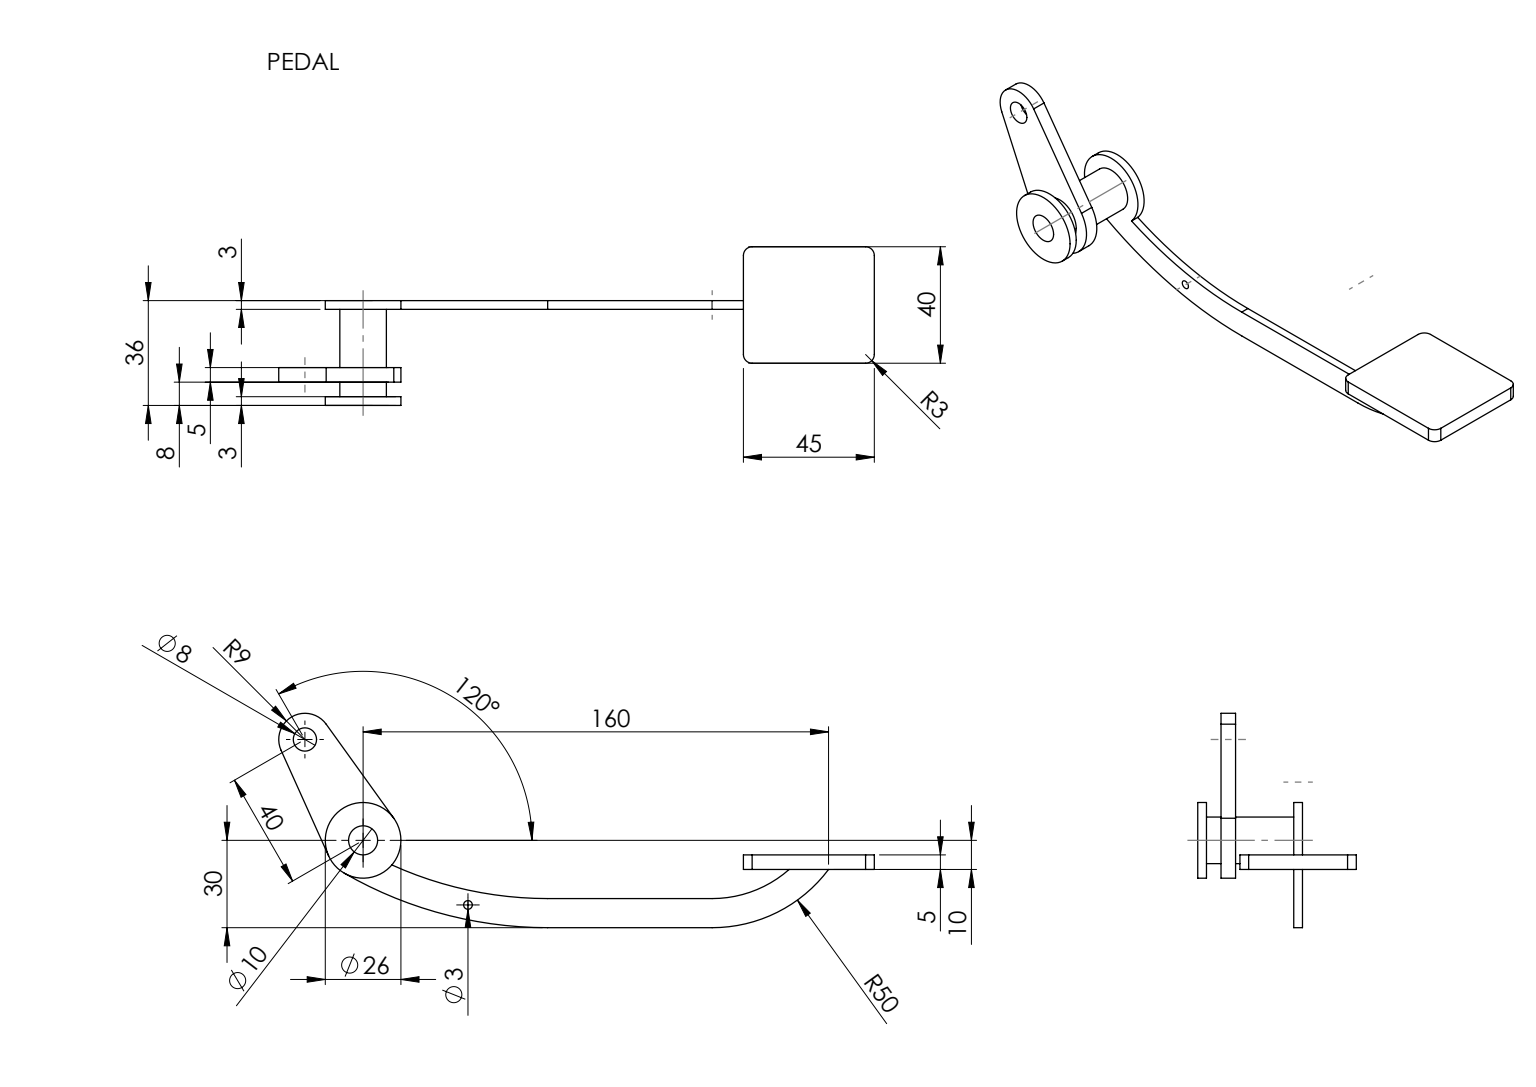
ISO-10303-21;
HEADER;
FILE_DESCRIPTION (('STEP AP214'),
    '1' );
FILE_NAME ('pedal.step',
    '2026-09-30T16:28:02',
    ( '' ),
    ( '' ),
    'SwSTEP 2.0',
    'SolidWorks 2026',
    '' );
FILE_SCHEMA (( 'AUTOMOTIVE_DESIGN' ));
ENDSEC;

DATA;
#42=STYLED_ITEM ( 'NONE', ( #6036 ), #28104 ) ;
#127=CYLINDRICAL_SURFACE ( 'NONE', #6337, 13.00000000000000178 ) ;
#249=ORIENTED_EDGE ( 'NONE', *, *, #10382, .F. ) ;
#257=ORIENTED_EDGE ( 'NONE', *, *, #15684, .T. ) ;
#314=VERTEX_POINT ( 'NONE', #24094 ) ;
#379=VERTEX_POINT ( 'NONE', #12319 ) ;
#383=DIRECTION ( 'NONE',  ( 1.000000000000000000, 2.891205793294675861E-16, 0.000000000000000000 ) ) ;
#395=DIRECTION ( 'NONE',  ( 1.000000000000000000, 0.000000000000000000, -0.000000000000000000 ) ) ;
#434=ORIENTED_EDGE ( 'NONE', *, *, #645, .T. ) ;
#454=CARTESIAN_POINT ( 'NONE',  ( 63.44486372867152824, 109.8897274573438096, -186.4312945166758482 ) ) ;
#465=CARTESIAN_POINT ( 'NONE',  ( 130.7287565553229456, -4.999999999999983125, 3.500000000000003109 ) ) ;
#488=CIRCLE ( 'NONE', #12639, 4.000000000000000000 ) ;
#489=EDGE_CURVE ( 'NONE', #20712, #9080, #7254, .T. ) ;
#529=MECHANICAL_DESIGN_GEOMETRIC_PRESENTATION_REPRESENTATION('',(#42),#25882);
#533=ORIENTED_EDGE ( 'NONE', *, *, #15684, .F. ) ;
#589=ORIENTED_EDGE ( 'NONE', *, *, #23254, .T. ) ;
#603=CARTESIAN_POINT ( 'NONE',  ( 34.54859390953723874, -22.18451583373416014, -18.00000000000000000 ) ) ;
#632=CIRCLE ( 'NONE', #16698, 4.000000000000000000 ) ;
#645=EDGE_CURVE ( 'NONE', #3816, #11753, #19590, .T. ) ;
#657=CARTESIAN_POINT ( 'NONE',  ( -16.00000000000017053, 34.64101615137744972, 4.999999999999998224 ) ) ;
#669=AXIS2_PLACEMENT_3D ( 'NONE', #29808, #9407, #6697 ) ;
#677=DIRECTION ( 'NONE',  ( -1.000000000000000000, 0.000000000000000000, -0.000000000000000000 ) ) ;
#683=ADVANCED_FACE ( 'NONE', ( #15154 ), #3431, .F. ) ;
#692=LINE ( 'NONE', #7853, #7318 ) ;
#721=DIRECTION ( 'NONE',  ( -1.000000000000000000, 0.000000000000000000, -0.000000000000000000 ) ) ;
#742=PLANE ( 'NONE',  #29494 ) ;
#762=ORIENTED_EDGE ( 'NONE', *, *, #27042, .F. ) ;
#821=ORIENTED_EDGE ( 'NONE', *, *, #21331, .F. ) ;
#837=ORIENTED_EDGE ( 'NONE', *, *, #25148, .F. ) ;
#841=DIRECTION ( 'NONE',  ( 0.000000000000000000, 0.000000000000000000, 1.000000000000000000 ) ) ;
#844=DIRECTION ( 'NONE',  ( 0.000000000000000000, 0.000000000000000000, 1.000000000000000000 ) ) ;
#867=CARTESIAN_POINT ( 'NONE',  ( 175.7287565553229456, -9.999999999999971578, -33.50000000000000000 ) ) ;
#928=EDGE_LOOP ( 'NONE', ( #6024, #1799, #821, #18334 ) ) ;
#930=VERTEX_POINT ( 'NONE', #27092 ) ;
#984=DIRECTION ( 'NONE',  ( 0.000000000000000000, 0.000000000000000000, 1.000000000000000000 ) ) ;
#988=AXIS2_PLACEMENT_3D ( 'NONE', #21614, #17036, #3172 ) ;
#995=EDGE_CURVE ( 'NONE', #29111, #15160, #24932, .T. ) ;
#999=DIRECTION ( 'NONE',  ( 0.000000000000000000, 0.000000000000000000, 1.000000000000000000 ) ) ;
#1037=DIRECTION ( 'NONE',  ( 0.000000000000000000, 0.000000000000000000, 1.000000000000000000 ) ) ;
#1038=ADVANCED_FACE ( 'NONE', ( #7466, #11728, #5018 ), #7170, .F. ) ;
#1062=AXIS2_PLACEMENT_3D ( 'NONE', #26492, #7854, #7556 ) ;
#1064=DIRECTION ( 'NONE',  ( 0.000000000000000000, 0.000000000000000000, 1.000000000000000000 ) ) ;
#1066=VECTOR ( 'NONE', #30185, 1000.000000000000114 ) ;
#1067=CARTESIAN_POINT ( 'NONE',  ( 172.7287565553229456, -9.999999999999971578, 3.500000000000003109 ) ) ;
#1093=DIRECTION ( 'NONE',  ( 1.000000000000000000, 1.226925503391459091E-16, -0.000000000000000000 ) ) ;
#1117=DIRECTION ( 'NONE',  ( 1.000000000000000000, 0.000000000000000000, 0.000000000000000000 ) ) ;
#1139=LINE ( 'NONE', #10420, #27314 ) ;
#1172=EDGE_LOOP ( 'NONE', ( #6000, #17827, #10475, #18155 ) ) ;
#1176=CARTESIAN_POINT ( 'NONE',  ( 63.44486372867152824, -29.99999999999998934, -186.4312945166758482 ) ) ;
#1182=AXIS2_PLACEMENT_3D ( 'NONE', #27480, #22255, #20556 ) ;
#1207=EDGE_CURVE ( 'NONE', #30188, #16793, #8258, .T. ) ;
#1274=LINE ( 'NONE', #5847, #25670 ) ;
#1287=AXIS2_PLACEMENT_3D ( 'NONE', #24642, #17167, #24199 ) ;
#1295=DIRECTION ( 'NONE',  ( -0.000000000000000000, -0.000000000000000000, 1.000000000000000000 ) ) ;
#1301=EDGE_LOOP ( 'NONE', ( #27535, #10792, #12334, #6173 ) ) ;
#1318=EDGE_CURVE ( 'NONE', #29111, #22823, #24707, .T. ) ;
#1338=VERTEX_POINT ( 'NONE', #29162 ) ;
#1360=VECTOR ( 'NONE', #4468, 1000.000000000000000 ) ;
#1406=DIRECTION ( 'NONE',  ( -0.000000000000000000, 0.000000000000000000, 1.000000000000000000 ) ) ;
#1410=ADVANCED_FACE ( 'NONE', ( #20402 ), #3946, .F. ) ;
#1444=EDGE_LOOP ( 'NONE', ( #23395, #23568, #5169, #4778 ) ) ;
#1454=EDGE_CURVE ( 'NONE', #14318, #9080, #6531, .T. ) ;
#1467=VECTOR ( 'NONE', #2467, 1000.000000000000000 ) ;
#1477=ADVANCED_FACE ( 'NONE', ( #11100 ), #17961, .T. ) ;
#1505=VECTOR ( 'NONE', #21440, 1000.000000000000000 ) ;
#1511=DIRECTION ( 'NONE',  ( 1.000000000000000000, 0.000000000000000000, -0.000000000000000000 ) ) ;
#1552=EDGE_CURVE ( 'NONE', #11816, #24750, #26302, .T. ) ;
#1575=PRODUCT ( 'pedal', 'pedal', '', ( #24431 ) ) ;
#1581=EDGE_CURVE ( 'NONE', #6067, #24792, #488, .T. ) ;
#1630=EDGE_CURVE ( 'NONE', #27716, #17672, #28296, .T. ) ;
#1648=CARTESIAN_POINT ( 'NONE',  ( 175.7287565553229456, -4.999999999999970690, 3.500000000000003109 ) ) ;
#1652=ORIENTED_EDGE ( 'NONE', *, *, #2676, .T. ) ;
#1687=ADVANCED_FACE ( 'NONE', ( #20851 ), #30235, .T. ) ;
#1715=CARTESIAN_POINT ( 'NONE',  ( -5.000000000000000000, 0.000000000000000000, -18.00000000000000000 ) ) ;
#1745=CARTESIAN_POINT ( 'NONE',  ( 2.698458740408370316E-15, -10.00000000000001776, 0.000000000000000000 ) ) ;
#1760=ORIENTED_EDGE ( 'NONE', *, *, #27900, .F. ) ;
#1762=EDGE_CURVE ( 'NONE', #930, #1338, #12665, .T. ) ;
#1799=ORIENTED_EDGE ( 'NONE', *, *, #17707, .F. ) ;
#1803=EDGE_CURVE ( 'NONE', #24538, #8805, #5361, .T. ) ;
#1858=CARTESIAN_POINT ( 'NONE',  ( 0.000000000000000000, 0.000000000000000000, 4.999999999999997335 ) ) ;
#1899=LINE ( 'NONE', #3878, #27335 ) ;
#1936=EDGE_CURVE ( 'NONE', #13441, #25891, #3908, .T. ) ;
#1968=EDGE_LOOP ( 'NONE', ( #25207, #6076, #3223, #29181, #3649 ) ) ;
#2005=DIRECTION ( 'NONE',  ( -0.000000000000000000, -0.000000000000000000, -1.000000000000000000 ) ) ;
#2022=CARTESIAN_POINT ( 'NONE',  ( 37.54859390953724585, -22.18451583373416014, -18.00000000000000000 ) ) ;
#2035=DIRECTION ( 'NONE',  ( 2.698458740408365879E-16, -1.000000000000000000, 0.000000000000000000 ) ) ;
#2043=CARTESIAN_POINT ( 'NONE',  ( -13.00000000000000178, 1.592040838891559293E-15, 15.00000000000000000 ) ) ;
#2051=ORIENTED_EDGE ( 'NONE', *, *, #1762, .F. ) ;
#2090=CYLINDRICAL_SURFACE ( 'NONE', #3703, 8.000000000000000000 ) ;
#2095=CARTESIAN_POINT ( 'NONE',  ( -12.69484042717385464, 39.89788248176327556, 4.999999999999998224 ) ) ;
#2097=DIRECTION ( 'NONE',  ( -0.000000000000000000, 0.000000000000000000, 1.000000000000000000 ) ) ;
#2162=FACE_OUTER_BOUND ( 'NONE', #11468, .T. ) ;
#2193=CARTESIAN_POINT ( 'NONE',  ( 146.4575131106458912, -9.999999999999976907, -15.00000000000000000 ) ) ;
#2230=VECTOR ( 'NONE', #14958, 1000.000000000000000 ) ;
#2256=CIRCLE ( 'NONE', #6137, 1.500000000000001332 ) ;
#2276=AXIS2_PLACEMENT_3D ( 'NONE', #10583, #20335, #6166 ) ;
#2297=AXIS2_PLACEMENT_3D ( 'NONE', #25842, #21241, #11775 ) ;
#2312=CARTESIAN_POINT ( 'NONE',  ( 8.000000000000000000, 9.797174393178825657E-16, -15.00000000000000355 ) ) ;
#2329=ORIENTED_EDGE ( 'NONE', *, *, #11651, .T. ) ;
#2360=CARTESIAN_POINT ( 'NONE',  ( 0.000000000000000000, 0.000000000000000000, 9.999999999999998224 ) ) ;
#2378=DIRECTION ( 'NONE',  ( 1.000000000000000000, 0.000000000000000000, 0.000000000000000000 ) ) ;
#2383=CARTESIAN_POINT ( 'NONE',  ( 13.00000000000000178, 0.000000000000000000, 15.00000000000000000 ) ) ;
#2417=DIRECTION ( 'NONE',  ( -1.000000000000000000, 0.000000000000000000, 0.000000000000000000 ) ) ;
#2429=AXIS2_PLACEMENT_3D ( 'NONE', #8510, #15976, #10947 ) ;
#2446=DIRECTION ( 'NONE',  ( 1.000000000000000000, 2.891205793294675861E-16, 0.000000000000000000 ) ) ;
#2453=AXIS2_PLACEMENT_3D ( 'NONE', #15182, #26515, #5445 ) ;
#2455=DIRECTION ( 'NONE',  ( 2.908569913943825554E-16, -1.000000000000000000, 0.000000000000000000 ) ) ;
#2467=DIRECTION ( 'NONE',  ( 6.938893903907227392E-16, -0.000000000000000000, 1.000000000000000000 ) ) ;
#2471=VERTEX_POINT ( 'NONE', #22637 ) ;
#2540=CARTESIAN_POINT ( 'NONE',  ( -8.000000000000000000, 0.000000000000000000, 9.999999999999998224 ) ) ;
#2571=DIRECTION ( 'NONE',  ( -0.000000000000000000, 0.000000000000000000, 1.000000000000000000 ) ) ;
#2646=CARTESIAN_POINT ( 'NONE',  ( 36.04859390953723874, -22.18451583373416014, -36.50100000000000477 ) ) ;
#2649=EDGE_CURVE ( 'NONE', #6067, #14522, #9326, .T. ) ;
#2676=EDGE_CURVE ( 'NONE', #10978, #24619, #21087, .T. ) ;
#2706=VERTEX_POINT ( 'NONE', #9172 ) ;
#2716=ADVANCED_FACE ( 'NONE', ( #30009 ), #23229, .T. ) ;
#2724=CIRCLE ( 'NONE', #18374, 9.000000000000007105 ) ;
#2728=ORIENTED_EDGE ( 'NONE', *, *, #18823, .T. ) ;
#2740=ORIENTED_EDGE ( 'NONE', *, *, #23334, .T. ) ;
#2743=DIRECTION ( 'NONE',  ( -0.000000000000000000, 0.000000000000000000, 1.000000000000000000 ) ) ;
#2745=CIRCLE ( 'NONE', #1287, 8.000000000000000000 ) ;
#2785=ORIENTED_EDGE ( 'NONE', *, *, #16826, .F. ) ;
#2808=ORIENTED_EDGE ( 'NONE', *, *, #1630, .F. ) ;
#2838=CARTESIAN_POINT ( 'NONE',  ( 0.000000000000000000, 0.000000000000000000, 18.00000000000000000 ) ) ;
#2877=CARTESIAN_POINT ( 'NONE',  ( 0.000000000000000000, 0.000000000000000000, -15.00000000000000000 ) ) ;
#2960=CYLINDRICAL_SURFACE ( 'NONE', #12674, 49.99999999999998579 ) ;
#2962=EDGE_LOOP ( 'NONE', ( #16694, #21576, #18341, #27834, #8161, #7484, #19166, #22520, #25922, #589 ) ) ;
#2976=CARTESIAN_POINT ( 'NONE',  ( 133.7287565553229456, -9.999999999999982236, 3.500000000000003109 ) ) ;
#2978=VECTOR ( 'NONE', #6080, 1000.000000000000000 ) ;
#2985=DIRECTION ( 'NONE',  ( 0.000000000000000000, 0.000000000000000000, -1.000000000000000000 ) ) ;
#2997=DIRECTION ( 'NONE',  ( -0.000000000000000000, -0.000000000000000000, -1.000000000000000000 ) ) ;
#3000=DIRECTION ( 'NONE',  ( -1.000000000000000000, 0.000000000000000000, 0.000000000000000000 ) ) ;
#3053=AXIS2_PLACEMENT_3D ( 'NONE', #23053, #2005, #29522 ) ;
#3079=EDGE_LOOP ( 'NONE', ( #2051, #17623, #29281, #13153, #6344, #2329, #5999, #6858, #17247, #29588 ) ) ;
#3111=FACE_OUTER_BOUND ( 'NONE', #29817, .T. ) ;
#3119=VERTEX_POINT ( 'NONE', #7615 ) ;
#3150=PLANE ( 'NONE',  #13903 ) ;
#3172=DIRECTION ( 'NONE',  ( -1.000000000000000000, 0.000000000000000000, 0.000000000000000000 ) ) ;
#3209=( GEOMETRIC_REPRESENTATION_CONTEXT ( 3 ) GLOBAL_UNCERTAINTY_ASSIGNED_CONTEXT ( ( #25987 ) ) GLOBAL_UNIT_ASSIGNED_CONTEXT ( ( #18544, #16247, #22987 ) ) REPRESENTATION_CONTEXT ( 'NONE', 'WORKASPACE' ) );
#3222=CIRCLE ( 'NONE', #5140, 13.00000000000000178 ) ;
#3223=ORIENTED_EDGE ( 'NONE', *, *, #26222, .T. ) ;
#3230=ORIENTED_EDGE ( 'NONE', *, *, #20276, .F. ) ;
#3234=CIRCLE ( 'NONE', #9538, 1.500000000000001332 ) ;
#3251=ORIENTED_EDGE ( 'NONE', *, *, #7811, .F. ) ;
#3268=DIRECTION ( 'NONE',  ( -1.000000000000000000, 0.000000000000000000, 0.000000000000000000 ) ) ;
#3286=CARTESIAN_POINT ( 'NONE',  ( 8.000000000000000000, 9.797174393178825657E-16, 4.999999999999997335 ) ) ;
#3292=DIRECTION ( 'NONE',  ( 1.000000000000000000, 0.000000000000000000, 0.000000000000000000 ) ) ;
#3338=ORIENTED_EDGE ( 'NONE', *, *, #11651, .F. ) ;
#3345=DIRECTION ( 'NONE',  ( 0.000000000000000000, 0.000000000000000000, 1.000000000000000000 ) ) ;
#3395=FACE_OUTER_BOUND ( 'NONE', #18625, .T. ) ;
#3418=FACE_OUTER_BOUND ( 'NONE', #14283, .T. ) ;
#3428=AXIS2_PLACEMENT_3D ( 'NONE', #10745, #844, #28962 ) ;
#3431=CYLINDRICAL_SURFACE ( 'NONE', #6294, 1.500000000000001332 ) ;
#3483=EDGE_CURVE ( 'NONE', #10508, #28576, #14252, .T. ) ;
#3492=CARTESIAN_POINT ( 'NONE',  ( -24.00000000000017053, 34.64101615137744972, 4.999999999999998224 ) ) ;
#3500=DIRECTION ( 'NONE',  ( 1.000000000000000000, 0.000000000000000000, -0.000000000000000000 ) ) ;
#3552=ORIENTED_EDGE ( 'NONE', *, *, #27900, .T. ) ;
#3604=EDGE_CURVE ( 'NONE', #12245, #8342, #21890, .T. ) ;
#3618=CARTESIAN_POINT ( 'NONE',  ( 63.44486372867152824, -29.99999999999998934, -15.00000000000000000 ) ) ;
#3643=FACE_OUTER_BOUND ( 'NONE', #1172, .T. ) ;
#3649=ORIENTED_EDGE ( 'NONE', *, *, #26284, .T. ) ;
#3661=EDGE_LOOP ( 'NONE', ( #23442, #28271, #21830, #25501 ) ) ;
#3668=DIRECTION ( 'NONE',  ( 1.000000000000000000, 0.000000000000000000, 0.000000000000000000 ) ) ;
#3678=EDGE_CURVE ( 'NONE', #19490, #2471, #692, .T. ) ;
#3698=AXIS2_PLACEMENT_3D ( 'NONE', #26593, #28769, #19699 ) ;
#3703=AXIS2_PLACEMENT_3D ( 'NONE', #11367, #2997, #12273 ) ;
#3747=SURFACE_STYLE_USAGE ( .BOTH. , #24352 ) ;
#3758=DIRECTION ( 'NONE',  ( 2.908569913943825554E-16, -1.000000000000000000, 0.000000000000000000 ) ) ;
#3791=FACE_OUTER_BOUND ( 'NONE', #25500, .T. ) ;
#3798=CARTESIAN_POINT ( 'NONE',  ( 5.000000000000000000, 6.123233995736766282E-16, 18.00000000000000000 ) ) ;
#3816=VERTEX_POINT ( 'NONE', #30018 ) ;
#3831=CIRCLE ( 'NONE', #22829, 9.000000000000007105 ) ;
#3835=DIRECTION ( 'NONE',  ( 0.4108911781748706971, -0.9116843969807022496, 0.000000000000000000 ) ) ;
#3878=CARTESIAN_POINT ( 'NONE',  ( 146.4575131106458912, -10.00000000000000178, -17.99999999999998934 ) ) ;
#3893=VERTEX_POINT ( 'NONE', #17856 ) ;
#3908=LINE ( 'NONE', #22979, #11680 ) ;
#3946=CYLINDRICAL_SURFACE ( 'NONE', #2429, 4.000000000000000000 ) ;
#3948=CARTESIAN_POINT ( 'NONE',  ( 175.7287565553229456, -9.999999999999971578, 3.500000000000003109 ) ) ;
#3973=DIRECTION ( 'NONE',  ( 0.000000000000000000, 0.000000000000000000, 1.000000000000000000 ) ) ;
#3991=CARTESIAN_POINT ( 'NONE',  ( -11.85189716074912880, -5.341585316273318895, 4.999999999999998224 ) ) ;
#4091=VECTOR ( 'NONE', #4105, 1000.000000000000000 ) ;
#4099=ADVANCED_FACE ( 'NONE', ( #25768 ), #12165, .F. ) ;
#4105=DIRECTION ( 'NONE',  ( 1.000000000000000000, 2.698458740408367851E-16, 0.000000000000000000 ) ) ;
#4153=DIRECTION ( 'NONE',  ( 1.000000000000000000, 2.698458740408365879E-16, 0.000000000000000000 ) ) ;
#4169=ORIENTED_EDGE ( 'NONE', *, *, #15331, .T. ) ;
#4172=AXIS2_PLACEMENT_3D ( 'NONE', #2646, #9640, #18661 ) ;
#4199=ADVANCED_FACE ( 'NONE', ( #28398 ), #26230, .T. ) ;
#4203=AXIS2_PLACEMENT_3D ( 'NONE', #2838, #999, #3292 ) ;
#4246=LINE ( 'NONE', #3948, #5558 ) ;
#4251=PRODUCT_DEFINITION_SHAPE ( 'NONE', 'NONE',  #15091 ) ;
#4285=ORIENTED_EDGE ( 'NONE', *, *, #23334, .F. ) ;
#4320=FACE_OUTER_BOUND ( 'NONE', #12707, .T. ) ;
#4390=CARTESIAN_POINT ( 'NONE',  ( -8.000000000000000000, 0.000000000000000000, 18.00000000000000000 ) ) ;
#4417=CARTESIAN_POINT ( 'NONE',  ( 63.44486372867152824, 109.8897274573438096, -17.99999999999998934 ) ) ;
#4435=EDGE_CURVE ( 'NONE', #8020, #8342, #12218, .T. ) ;
#4468=DIRECTION ( 'NONE',  ( 0.000000000000000000, 0.000000000000000000, 1.000000000000000000 ) ) ;
#4506=VECTOR ( 'NONE', #3345, 1000.000000000000000 ) ;
#4570=AXIS2_PLACEMENT_3D ( 'NONE', #25153, #8512, #6081 ) ;
#4582=ORIENTED_EDGE ( 'NONE', *, *, #995, .F. ) ;
#4668=AXIS2_PLACEMENT_3D ( 'NONE', #1648, #10469, #15199 ) ;
#4718=CYLINDRICAL_SURFACE ( 'NONE', #19500, 139.8897274573438096 ) ;
#4723=VERTEX_POINT ( 'NONE', #18433 ) ;
#4742=ORIENTED_EDGE ( 'NONE', *, *, #27938, .F. ) ;
#4749=ORIENTED_EDGE ( 'NONE', *, *, #9869, .F. ) ;
#4750=DIRECTION ( 'NONE',  ( -1.000000000000000000, -1.226925503391459091E-16, 0.000000000000000000 ) ) ;
#4776=DIRECTION ( 'NONE',  ( 1.000000000000000000, 0.000000000000000000, 0.000000000000000000 ) ) ;
#4778=ORIENTED_EDGE ( 'NONE', *, *, #10769, .T. ) ;
#4840=EDGE_LOOP ( 'NONE', ( #13329, #13034 ) ) ;
#4844=CARTESIAN_POINT ( 'NONE',  ( 0.000000000000000000, 0.000000000000000000, 4.999999999999998224 ) ) ;
#4849=DIRECTION ( 'NONE',  ( 0.000000000000000000, 0.000000000000000000, 1.000000000000000000 ) ) ;
#4867=DIRECTION ( 'NONE',  ( 1.000000000000000000, 0.000000000000000000, -0.000000000000000000 ) ) ;
#4884=VERTEX_POINT ( 'NONE', #5605 ) ;
#4900=DIRECTION ( 'NONE',  ( -0.000000000000000000, 0.000000000000000000, 1.000000000000000000 ) ) ;
#4906=ORIENTED_EDGE ( 'NONE', *, *, #20615, .T. ) ;
#4924=EDGE_LOOP ( 'NONE', ( #15642, #20260, #22893, #5865 ) ) ;
#4928=DIRECTION ( 'NONE',  ( -0.000000000000000000, 0.000000000000000000, 1.000000000000000000 ) ) ;
#4943=VERTEX_POINT ( 'NONE', #3618 ) ;
#4945=CIRCLE ( 'NONE', #6854, 13.00000000000000178 ) ;
#4949=EDGE_CURVE ( 'NONE', #6425, #27841, #26219, .T. ) ;
#4974=ORIENTED_EDGE ( 'NONE', *, *, #489, .T. ) ;
#4980=EDGE_CURVE ( 'NONE', #9455, #314, #8027, .T. ) ;
#4986=CARTESIAN_POINT ( 'NONE',  ( -20.00000000000017053, 34.64101615137744972, 4.999999999999998224 ) ) ;
#4987=ORIENTED_EDGE ( 'NONE', *, *, #28241, .T. ) ;
#4999=FACE_OUTER_BOUND ( 'NONE', #3079, .T. ) ;
#5018=FACE_OUTER_BOUND ( 'NONE', #2962, .T. ) ;
#5056=ORIENTED_EDGE ( 'NONE', *, *, #9583, .T. ) ;
#5063=CARTESIAN_POINT ( 'NONE',  ( -12.69484042717385464, 39.89788248176327556, 4.999999999999998224 ) ) ;
#5111=AXIS2_PLACEMENT_3D ( 'NONE', #25524, #8881, #18193 ) ;
#5140=AXIS2_PLACEMENT_3D ( 'NONE', #11668, #8632, #17933 ) ;
#5165=LINE ( 'NONE', #18748, #26250 ) ;
#5169=ORIENTED_EDGE ( 'NONE', *, *, #2649, .T. ) ;
#5192=EDGE_CURVE ( 'NONE', #27841, #4723, #20039, .T. ) ;
#5255=DIRECTION ( 'NONE',  ( 1.000000000000000000, -1.840388255087189623E-16, 0.000000000000000000 ) ) ;
#5301=CARTESIAN_POINT ( 'NONE',  ( 37.54859390953724585, -22.18451583373416014, -36.50100000000000477 ) ) ;
#5317=DIRECTION ( 'NONE',  ( 1.000000000000000000, 0.000000000000000000, 0.000000000000000000 ) ) ;
#5319=DIRECTION ( 'NONE',  ( 2.908569913943825554E-16, -1.000000000000000000, 0.000000000000000000 ) ) ;
#5325=CARTESIAN_POINT ( 'NONE',  ( 133.7287565553229456, -4.999999999999982236, 3.500000000000003109 ) ) ;
#5329=PLANE ( 'NONE',  #12197 ) ;
#5361=CIRCLE ( 'NONE', #2453, 5.000000000000000000 ) ;
#5375=LINE ( 'NONE', #5063, #29555 ) ;
#5394=CARTESIAN_POINT ( 'NONE',  ( 130.7287565553229456, -9.999999999999982236, 0.5000000000000052180 ) ) ;
#5397=CARTESIAN_POINT ( 'NONE',  ( 130.7287565553229456, -9.999999999999982236, 3.500000000000003109 ) ) ;
#5404=ORIENTED_EDGE ( 'NONE', *, *, #24061, .T. ) ;
#5422=CYLINDRICAL_SURFACE ( 'NONE', #1062, 4.000000000000000000 ) ;
#5435=CARTESIAN_POINT ( 'NONE',  ( 0.000000000000000000, 0.000000000000000000, 0.000000000000000000 ) ) ;
#5445=DIRECTION ( 'NONE',  ( 1.000000000000000000, 0.000000000000000000, 0.000000000000000000 ) ) ;
#5452=DIRECTION ( 'NONE',  ( -0.000000000000000000, -0.000000000000000000, 1.000000000000000000 ) ) ;
#5455=CARTESIAN_POINT ( 'NONE',  ( 9.884967449281287344, -8.443187699361503817, -15.00000000000000000 ) ) ;
#5466=ADVANCED_FACE ( 'NONE', ( #29108 ), #5422, .F. ) ;
#5473=ADVANCED_FACE ( 'NONE', ( #17163 ), #12726, .T. ) ;
#5500=EDGE_CURVE ( 'NONE', #29186, #16077, #4945, .T. ) ;
#5551=EDGE_CURVE ( 'NONE', #3893, #2706, #7325, .T. ) ;
#5558=VECTOR ( 'NONE', #15373, 1000.000000000000000 ) ;
#5605=CARTESIAN_POINT ( 'NONE',  ( 172.7287565553229456, -4.999999999999971578, -36.50000000000000711 ) ) ;
#5666=CIRCLE ( 'NONE', #9540, 8.000000000000000000 ) ;
#5674=LINE ( 'NONE', #8094, #2230 ) ;
#5716=ADVANCED_FACE ( 'NONE', ( #29264 ), #20193, .F. ) ;
#5757=DIRECTION ( 'NONE',  ( -1.000000000000000000, 1.840388255087189623E-16, 0.000000000000000000 ) ) ;
#5844=FACE_OUTER_BOUND ( 'NONE', #1301, .T. ) ;
#5847=CARTESIAN_POINT ( 'NONE',  ( 34.54859390953723874, -22.18451583373416014, -36.50100000000000477 ) ) ;
#5865=ORIENTED_EDGE ( 'NONE', *, *, #26182, .F. ) ;
#5870=EDGE_LOOP ( 'NONE', ( #21744, #17723, #3552, #16571 ) ) ;
#5875=DIRECTION ( 'NONE',  ( 0.000000000000000000, 0.000000000000000000, 1.000000000000000000 ) ) ;
#5911=CARTESIAN_POINT ( 'NONE',  ( -20.00000000000017053, 34.64101615137744972, 9.999999999999998224 ) ) ;
#5931=ADVANCED_FACE ( 'NONE', ( #3111 ), #23862, .F. ) ;
#5999=ORIENTED_EDGE ( 'NONE', *, *, #21306, .T. ) ;
#6000=ORIENTED_EDGE ( 'NONE', *, *, #21516, .F. ) ;
#6019=ADVANCED_FACE ( 'NONE', ( #3395 ), #2960, .T. ) ;
#6022=EDGE_CURVE ( 'NONE', #314, #4943, #12385, .T. ) ;
#6024=ORIENTED_EDGE ( 'NONE', *, *, #29168, .F. ) ;
#6036=PRESENTATION_STYLE_ASSIGNMENT (( #3747 ) ) ;
#6042=LINE ( 'NONE', #20075, #17224 ) ;
#6067=VERTEX_POINT ( 'NONE', #657 ) ;
#6076=ORIENTED_EDGE ( 'NONE', *, *, #26828, .T. ) ;
#6080=DIRECTION ( 'NONE',  ( -0.000000000000000000, -0.000000000000000000, -1.000000000000000000 ) ) ;
#6081=DIRECTION ( 'NONE',  ( 1.000000000000000000, 2.891205793294675861E-16, 0.000000000000000000 ) ) ;
#6111=DIRECTION ( 'NONE',  ( -0.000000000000000000, 0.000000000000000000, 1.000000000000000000 ) ) ;
#6137=AXIS2_PLACEMENT_3D ( 'NONE', #10592, #19901, #29268 ) ;
#6166=DIRECTION ( 'NONE',  ( 1.000000000000000000, 2.891205793294675861E-16, 0.000000000000000000 ) ) ;
#6173=ORIENTED_EDGE ( 'NONE', *, *, #14540, .F. ) ;
#6236=DIRECTION ( 'NONE',  ( -0.000000000000000000, -0.000000000000000000, -1.000000000000000000 ) ) ;
#6276=FACE_OUTER_BOUND ( 'NONE', #8405, .T. ) ;
#6294=AXIS2_PLACEMENT_3D ( 'NONE', #22185, #1295, #21889 ) ;
#6304=DIRECTION ( 'NONE',  ( -0.000000000000000000, -0.000000000000000000, -1.000000000000000000 ) ) ;
#6321=CARTESIAN_POINT ( 'NONE',  ( 0.000000000000000000, 0.000000000000000000, 18.00000000000000000 ) ) ;
#6337=AXIS2_PLACEMENT_3D ( 'NONE', #4844, #25920, #18737 ) ;
#6344=ORIENTED_EDGE ( 'NONE', *, *, #26926, .T. ) ;
#6385=COLOUR_RGB ( '', 0.66274510, 0.83137255, 0.94901961) ;
#6417=LINE ( 'NONE', #18147, #21838 ) ;
#6425=VERTEX_POINT ( 'NONE', #2022 ) ;
#6448=CIRCLE ( 'NONE', #16165, 129.8897274573438381 ) ;
#6450=PLANE ( 'NONE',  #28423 ) ;
#6531=LINE ( 'NONE', #4390, #7763 ) ;
#6638=CIRCLE ( 'NONE', #11497, 8.000000000000000000 ) ;
#6653=CARTESIAN_POINT ( 'NONE',  ( 0.000000000000000000, 0.000000000000000000, 15.00000000000000000 ) ) ;
#6697=DIRECTION ( 'NONE',  ( -1.000000000000000000, 0.000000000000000000, 0.000000000000000000 ) ) ;
#6711=VECTOR ( 'NONE', #26813, 1000.000000000000000 ) ;
#6796=AXIS2_PLACEMENT_3D ( 'NONE', #23766, #16272, #2417 ) ;
#6811=ORIENTED_EDGE ( 'NONE', *, *, #1803, .T. ) ;
#6822=ORIENTED_EDGE ( 'NONE', *, *, #26182, .T. ) ;
#6837=CARTESIAN_POINT ( 'NONE',  ( 0.000000000000000000, 0.000000000000000000, 18.00000000000000000 ) ) ;
#6839=ORIENTED_EDGE ( 'NONE', *, *, #2649, .F. ) ;
#6840=VECTOR ( 'NONE', #7687, 1000.000000000000000 ) ;
#6854=AXIS2_PLACEMENT_3D ( 'NONE', #8148, #24195, #10430 ) ;
#6858=ORIENTED_EDGE ( 'NONE', *, *, #7905, .T. ) ;
#6933=CARTESIAN_POINT ( 'NONE',  ( 10.55189716074911921, 7.593251366112848899, 9.999999999999998224 ) ) ;
#7036=FACE_OUTER_BOUND ( 'NONE', #5870, .T. ) ;
#7103=CARTESIAN_POINT ( 'NONE',  ( 0.000000000000000000, 0.000000000000000000, 15.00000000000000000 ) ) ;
#7109=CARTESIAN_POINT ( 'NONE',  ( -8.000000000000000000, 0.000000000000000000, 4.999999999999997335 ) ) ;
#7132=CARTESIAN_POINT ( 'NONE',  ( -6.499999999999929834, -11.25833024919774239, -186.4312945166758482 ) ) ;
#7138=LINE ( 'NONE', #16437, #4091 ) ;
#7140=DIRECTION ( 'NONE',  ( 1.000000000000000000, 2.891205793294675861E-16, 0.000000000000000000 ) ) ;
#7145=CARTESIAN_POINT ( 'NONE',  ( 0.000000000000000000, 0.000000000000000000, 18.00000000000000000 ) ) ;
#7170=PLANE ( 'NONE',  #9696 ) ;
#7212=CARTESIAN_POINT ( 'NONE',  ( 0.000000000000000000, 0.000000000000000000, 4.999999999999998224 ) ) ;
#7239=EDGE_LOOP ( 'NONE', ( #9386, #2785, #25854, #20739 ) ) ;
#7254=CIRCLE ( 'NONE', #9169, 8.000000000000000000 ) ;
#7280=CARTESIAN_POINT ( 'NONE',  ( 133.7287565553229172, -4.999999999999982236, -36.50000000000000711 ) ) ;
#7305=DIRECTION ( 'NONE',  ( -1.000000000000000000, -2.698458740408365879E-16, -0.000000000000000000 ) ) ;
#7312=VECTOR ( 'NONE', #11846, 1000.000000000000000 ) ;
#7318=VECTOR ( 'NONE', #5875, 1000.000000000000000 ) ;
#7325=CIRCLE ( 'NONE', #27350, 13.00000000000000178 ) ;
#7368=ADVANCED_FACE ( 'NONE', ( #8306, #8601, #20350 ), #17901, .F. ) ;
#7392=EDGE_LOOP ( 'NONE', ( #8815, #16678 ) ) ;
#7407=EDGE_CURVE ( 'NONE', #13148, #11753, #25541, .T. ) ;
#7414=CARTESIAN_POINT ( 'NONE',  ( 63.44486372867149981, -20.00000000000000355, -15.00000000000000000 ) ) ;
#7450=DIRECTION ( 'NONE',  ( -1.000000000000000000, 0.000000000000000000, 0.000000000000000000 ) ) ;
#7453=EDGE_LOOP ( 'NONE', ( #16835, #23521, #10468, #26752 ) ) ;
#7464=CARTESIAN_POINT ( 'NONE',  ( 5.000000000000000000, 6.123233995736766282E-16, -18.00000000000000000 ) ) ;
#7466=FACE_BOUND ( 'NONE', #8430, .T. ) ;
#7484=ORIENTED_EDGE ( 'NONE', *, *, #1630, .T. ) ;
#7538=CARTESIAN_POINT ( 'NONE',  ( -5.000000000000000000, 0.000000000000000000, 18.00000000000000000 ) ) ;
#7553=DIRECTION ( 'NONE',  ( -1.000000000000000000, -1.226925503391459338E-16, -0.000000000000000000 ) ) ;
#7556=DIRECTION ( 'NONE',  ( 1.000000000000000000, 0.000000000000000000, 0.000000000000000000 ) ) ;
#7588=DIRECTION ( 'NONE',  ( -2.698458740408365879E-16, 1.000000000000000000, -0.000000000000000000 ) ) ;
#7604=FACE_OUTER_BOUND ( 'NONE', #928, .T. ) ;
#7609=DIRECTION ( 'NONE',  ( 0.000000000000000000, 0.000000000000000000, 1.000000000000000000 ) ) ;
#7615=CARTESIAN_POINT ( 'NONE',  ( -28.20515957282649921, 30.94299554780361206, 4.999999999999998224 ) ) ;
#7626=DIRECTION ( 'NONE',  ( -0.000000000000000000, 0.000000000000000000, 1.000000000000000000 ) ) ;
#7635=VECTOR ( 'NONE', #28016, 1000.000000000000000 ) ;
#7651=CARTESIAN_POINT ( 'NONE',  ( 0.000000000000000000, 0.000000000000000000, -15.00000000000000000 ) ) ;
#7687=DIRECTION ( 'NONE',  ( -0.000000000000000000, -0.000000000000000000, -1.000000000000000000 ) ) ;
#7700=LINE ( 'NONE', #7414, #16851 ) ;
#7749=ORIENTED_EDGE ( 'NONE', *, *, #23254, .F. ) ;
#7763=VECTOR ( 'NONE', #9096, 1000.000000000000000 ) ;
#7791=CARTESIAN_POINT ( 'NONE',  ( 133.7287565553229456, -9.999999999999980460, 0.5000000000000029976 ) ) ;
#7808=DIRECTION ( 'NONE',  ( 0.000000000000000000, 0.000000000000000000, 1.000000000000000000 ) ) ;
#7811=EDGE_CURVE ( 'NONE', #19672, #20712, #12110, .T. ) ;
#7853=CARTESIAN_POINT ( 'NONE',  ( 13.00000000000000178, 0.000000000000000000, 15.00000000000000000 ) ) ;
#7854=DIRECTION ( 'NONE',  ( 0.000000000000000000, 0.000000000000000000, 1.000000000000000000 ) ) ;
#7875=ORIENTED_EDGE ( 'NONE', *, *, #4980, .F. ) ;
#7890=CARTESIAN_POINT ( 'NONE',  ( 36.04859390953723874, -22.18451583373416014, -18.00000000000000000 ) ) ;
#7905=EDGE_CURVE ( 'NONE', #10263, #29352, #6448, .T. ) ;
#7907=EDGE_CURVE ( 'NONE', #13441, #21824, #23886, .T. ) ;
#7913=DIRECTION ( 'NONE',  ( -0.8116843969807016057, -0.5840962589317576503, 0.000000000000000000 ) ) ;
#7958=CIRCLE ( 'NONE', #11381, 3.000000000000002665 ) ;
#7960=DIRECTION ( 'NONE',  ( 0.000000000000000000, 0.000000000000000000, 1.000000000000000000 ) ) ;
#7979=ORIENTED_EDGE ( 'NONE', *, *, #26926, .F. ) ;
#8019=ORIENTED_EDGE ( 'NONE', *, *, #12892, .T. ) ;
#8020=VERTEX_POINT ( 'NONE', #22329 ) ;
#8027=LINE ( 'NONE', #17336, #14162 ) ;
#8068=ADVANCED_FACE ( 'NONE', ( #3418 ), #22029, .T. ) ;
#8076=AXIS2_PLACEMENT_3D ( 'NONE', #5911, #11077, #22990 ) ;
#8094=CARTESIAN_POINT ( 'NONE',  ( 13.00000000000000178, 0.000000000000000000, 4.999999999999998224 ) ) ;
#8116=ORIENTED_EDGE ( 'NONE', *, *, #15206, .F. ) ;
#8148=CARTESIAN_POINT ( 'NONE',  ( 0.000000000000000000, 0.000000000000000000, 9.999999999999998224 ) ) ;
#8161=ORIENTED_EDGE ( 'NONE', *, *, #26597, .T. ) ;
#8167=DIRECTION ( 'NONE',  ( -2.908569913943825554E-16, 1.000000000000000000, -0.000000000000000000 ) ) ;
#8190=ORIENTED_EDGE ( 'NONE', *, *, #4435, .F. ) ;
#8248=DIRECTION ( 'NONE',  ( 1.000000000000000000, 2.908569913943825554E-16, -6.938893903907227392E-16 ) ) ;
#8251=CYLINDRICAL_SURFACE ( 'NONE', #3698, 13.00000000000000178 ) ;
#8258=CIRCLE ( 'NONE', #26821, 5.000000000000000000 ) ;
#8286=DIRECTION ( 'NONE',  ( -0.000000000000000000, -0.000000000000000000, -1.000000000000000000 ) ) ;
#8291=VECTOR ( 'NONE', #841, 1000.000000000000000 ) ;
#8306=FACE_OUTER_BOUND ( 'NONE', #20012, .T. ) ;
#8318=AXIS2_PLACEMENT_3D ( 'NONE', #28696, #12770, #22088 ) ;
#8322=ADVANCED_FACE ( 'NONE', ( #17874 ), #27404, .T. ) ;
#8337=LINE ( 'NONE', #20229, #25619 ) ;
#8342=VERTEX_POINT ( 'NONE', #13609 ) ;
#8344=FACE_OUTER_BOUND ( 'NONE', #12117, .T. ) ;
#8393=VECTOR ( 'NONE', #30227, 1000.000000000000000 ) ;
#8405=EDGE_LOOP ( 'NONE', ( #23698, #5404, #24121, #21265 ) ) ;
#8411=ORIENTED_EDGE ( 'NONE', *, *, #1207, .F. ) ;
#8417=ORIENTED_EDGE ( 'NONE', *, *, #27618, .T. ) ;
#8430=EDGE_LOOP ( 'NONE', ( #12068, #10052 ) ) ;
#8510=CARTESIAN_POINT ( 'NONE',  ( -20.00000000000017053, 34.64101615137744972, 4.999999999999998224 ) ) ;
#8512=DIRECTION ( 'NONE',  ( 2.908569913943825554E-16, -1.000000000000000000, 0.000000000000000000 ) ) ;
#8550=CIRCLE ( 'NONE', #8076, 4.000000000000000000 ) ;
#8593=DIRECTION ( 'NONE',  ( 1.000000000000000000, 0.000000000000000000, 0.000000000000000000 ) ) ;
#8601=FACE_BOUND ( 'NONE', #26626, .T. ) ;
#8602=VECTOR ( 'NONE', #28339, 1000.000000000000000 ) ;
#8620=ADVANCED_FACE ( 'NONE', ( #27214 ), #30121, .F. ) ;
#8632=DIRECTION ( 'NONE',  ( 0.000000000000000000, 0.000000000000000000, 1.000000000000000000 ) ) ;
#8676=DIRECTION ( 'NONE',  ( 1.000000000000000000, 2.891205793294675861E-16, 0.000000000000000000 ) ) ;
#8717=FACE_OUTER_BOUND ( 'NONE', #13862, .T. ) ;
#8805=VERTEX_POINT ( 'NONE', #7464 ) ;
#8815=ORIENTED_EDGE ( 'NONE', *, *, #15376, .T. ) ;
#8832=ORIENTED_EDGE ( 'NONE', *, *, #15588, .T. ) ;
#8840=DIRECTION ( 'NONE',  ( -1.000000000000000000, 0.000000000000000000, 0.000000000000000000 ) ) ;
#8852=EDGE_LOOP ( 'NONE', ( #15720, #1652, #533, #8875 ) ) ;
#8865=EDGE_CURVE ( 'NONE', #11598, #14522, #632, .T. ) ;
#8875=ORIENTED_EDGE ( 'NONE', *, *, #3678, .F. ) ;
#8881=DIRECTION ( 'NONE',  ( 2.908569913943825554E-16, -1.000000000000000000, 0.000000000000000000 ) ) ;
#8911=AXIS2_PLACEMENT_3D ( 'NONE', #24217, #19170, #19466 ) ;
#8944=ORIENTED_EDGE ( 'NONE', *, *, #645, .F. ) ;
#8945=FACE_BOUND ( 'NONE', #4840, .T. ) ;
#9012=VECTOR ( 'NONE', #21357, 1000.000000000000000 ) ;
#9055=CARTESIAN_POINT ( 'NONE',  ( 172.7287565553229456, -9.999999999999971578, -33.50000000000000000 ) ) ;
#9080=VERTEX_POINT ( 'NONE', #29524 ) ;
#9084=ORIENTED_EDGE ( 'NONE', *, *, #13448, .F. ) ;
#9096=DIRECTION ( 'NONE',  ( -0.000000000000000000, -0.000000000000000000, -1.000000000000000000 ) ) ;
#9142=PLANE ( 'NONE',  #12659 ) ;
#9169=AXIS2_PLACEMENT_3D ( 'NONE', #16764, #24244, #29009 ) ;
#9172=CARTESIAN_POINT ( 'NONE',  ( 9.884967449281269580, -8.443187699361526910, -18.00000000000000000 ) ) ;
#9179=FACE_OUTER_BOUND ( 'NONE', #20250, .T. ) ;
#9216=SURFACE_SIDE_STYLE ('',( #13947 ) ) ;
#9324=ORIENTED_EDGE ( 'NONE', *, *, #23597, .F. ) ;
#9326=LINE ( 'NONE', #22942, #23775 ) ;
#9333=CYLINDRICAL_SURFACE ( 'NONE', #4172, 1.500000000000001332 ) ;
#9386=ORIENTED_EDGE ( 'NONE', *, *, #25069, .F. ) ;
#9407=DIRECTION ( 'NONE',  ( 0.000000000000000000, 0.000000000000000000, -1.000000000000000000 ) ) ;
#9455=VERTEX_POINT ( 'NONE', #28532 ) ;
#9538=AXIS2_PLACEMENT_3D ( 'NONE', #7890, #22390, #10783 ) ;
#9540=AXIS2_PLACEMENT_3D ( 'NONE', #1858, #6111, #24584 ) ;
#9548=DIRECTION ( 'NONE',  ( 0.000000000000000000, 0.000000000000000000, 1.000000000000000000 ) ) ;
#9576=LINE ( 'NONE', #28255, #13079 ) ;
#9583=EDGE_CURVE ( 'NONE', #11816, #930, #26213, .T. ) ;
#9628=EDGE_CURVE ( 'NONE', #27716, #16265, #24520, .T. ) ;
#9632=AXIS2_PLACEMENT_3D ( 'NONE', #19867, #14977, #3268 ) ;
#9640=DIRECTION ( 'NONE',  ( -0.000000000000000000, -0.000000000000000000, 1.000000000000000000 ) ) ;
#9647=DIRECTION ( 'NONE',  ( -0.000000000000000000, -0.000000000000000000, -1.000000000000000000 ) ) ;
#9696=AXIS2_PLACEMENT_3D ( 'NONE', #16460, #7609, #4867 ) ;
#9718=EDGE_CURVE ( 'NONE', #379, #26545, #29231, .T. ) ;
#9719=DIRECTION ( 'NONE',  ( -0.000000000000000000, -0.000000000000000000, -1.000000000000000000 ) ) ;
#9737=CARTESIAN_POINT ( 'NONE',  ( -20.00000000000017053, 34.64101615137744972, 9.999999999999998224 ) ) ;
#9833=CARTESIAN_POINT ( 'NONE',  ( 130.7287565553229172, -9.999999999999982236, -36.50000000000000711 ) ) ;
#9834=EDGE_CURVE ( 'NONE', #20421, #29352, #24860, .T. ) ;
#9836=DIRECTION ( 'NONE',  ( 0.000000000000000000, 0.000000000000000000, -1.000000000000000000 ) ) ;
#9860=ORIENTED_EDGE ( 'NONE', *, *, #1803, .F. ) ;
#9869=EDGE_CURVE ( 'NONE', #17672, #12245, #1899, .T. ) ;
#9872=ORIENTED_EDGE ( 'NONE', *, *, #7907, .F. ) ;
#9906=CARTESIAN_POINT ( 'NONE',  ( 175.7287565553229456, -4.999999999999970690, 0.5000000000000029976 ) ) ;
#9938=VERTEX_POINT ( 'NONE', #16211 ) ;
#9981=DIRECTION ( 'NONE',  ( 2.908569913943825554E-16, -1.000000000000000000, 0.000000000000000000 ) ) ;
#10032=EDGE_LOOP ( 'NONE', ( #9324, #4987, #10551, #1760 ) ) ;
#10052=ORIENTED_EDGE ( 'NONE', *, *, #23166, .F. ) ;
#10054=CYLINDRICAL_SURFACE ( 'NONE', #23311, 13.00000000000000178 ) ;
#10087=ORIENTED_EDGE ( 'NONE', *, *, #3483, .T. ) ;
#10091=CARTESIAN_POINT ( 'NONE',  ( 63.44486372867152824, -29.99999999999998934, -186.4312945166758482 ) ) ;
#10096=VERTEX_POINT ( 'NONE', #16810 ) ;
#10123=AXIS2_PLACEMENT_3D ( 'NONE', #13210, #27584, #20663 ) ;
#10134=CARTESIAN_POINT ( 'NONE',  ( 0.000000000000000000, 0.000000000000000000, -18.00000000000000000 ) ) ;
#10139=CARTESIAN_POINT ( 'NONE',  ( -16.00000000000017053, 34.64101615137744972, 9.999999999999998224 ) ) ;
#10190=VECTOR ( 'NONE', #8286, 1000.000000000000000 ) ;
#10193=DIRECTION ( 'NONE',  ( 0.000000000000000000, 0.000000000000000000, 1.000000000000000000 ) ) ;
#10195=AXIS2_PLACEMENT_3D ( 'NONE', #19171, #9548, #28230 ) ;
#10205=CARTESIAN_POINT ( 'NONE',  ( -20.00000000000017053, 34.64101615137744972, 4.999999999999998224 ) ) ;
#10220=CARTESIAN_POINT ( 'NONE',  ( 63.44486372867149981, -20.00000000000000355, -17.99999999999998934 ) ) ;
#10249=AXIS2_PLACEMENT_3D ( 'NONE', #28087, #4849, #14149 ) ;
#10258=DIRECTION ( 'NONE',  ( 1.000000000000000000, 0.000000000000000000, 0.000000000000000000 ) ) ;
#10263=VERTEX_POINT ( 'NONE', #18734 ) ;
#10280=DIRECTION ( 'NONE',  ( 1.000000000000000000, 0.000000000000000000, 0.000000000000000000 ) ) ;
#10309=EDGE_CURVE ( 'NONE', #24750, #3893, #18189, .T. ) ;
#10382=EDGE_CURVE ( 'NONE', #15160, #30082, #7138, .T. ) ;
#10409=CARTESIAN_POINT ( 'NONE',  ( 0.000000000000000000, 0.000000000000000000, 9.999999999999998224 ) ) ;
#10420=CARTESIAN_POINT ( 'NONE',  ( 10.55189716074911921, 7.593251366112848899, 4.999999999999998224 ) ) ;
#10430=DIRECTION ( 'NONE',  ( 1.000000000000000000, 0.000000000000000000, 0.000000000000000000 ) ) ;
#10446=DIRECTION ( 'NONE',  ( 1.000000000000000000, 0.000000000000000000, 0.000000000000000000 ) ) ;
#10468=ORIENTED_EDGE ( 'NONE', *, *, #21306, .F. ) ;
#10469=DIRECTION ( 'NONE',  ( -1.000000000000000000, -2.908569913943825554E-16, 0.000000000000000000 ) ) ;
#10475=ORIENTED_EDGE ( 'NONE', *, *, #17818, .F. ) ;
#10490=DIRECTION ( 'NONE',  ( 1.000000000000000000, 2.698458740408367851E-16, 0.000000000000000000 ) ) ;
#10505=CARTESIAN_POINT ( 'NONE',  ( 13.00000000000000178, 1.592040838891559293E-15, -15.00000000000000000 ) ) ;
#10508=VERTEX_POINT ( 'NONE', #21163 ) ;
#10510=CARTESIAN_POINT ( 'NONE',  ( -24.00000000000017053, 34.64101615137744972, 4.999999999999998224 ) ) ;
#10533=CARTESIAN_POINT ( 'NONE',  ( -11.85189716074912880, -5.341585316273318895, 4.999999999999998224 ) ) ;
#10551=ORIENTED_EDGE ( 'NONE', *, *, #11534, .T. ) ;
#10565=DIRECTION ( 'NONE',  ( 0.000000000000000000, 0.000000000000000000, 1.000000000000000000 ) ) ;
#10572=AXIS2_PLACEMENT_3D ( 'NONE', #25507, #18932, #20755 ) ;
#10583=CARTESIAN_POINT ( 'NONE',  ( 172.7287565553229456, -4.999999999999970690, -33.50000000000000000 ) ) ;
#10592=CARTESIAN_POINT ( 'NONE',  ( 36.04859390953723874, -22.18451583373416014, -18.00000000000000000 ) ) ;
#10619=DIRECTION ( 'NONE',  ( 1.000000000000000000, 0.000000000000000000, 0.000000000000000000 ) ) ;
#10651=CYLINDRICAL_SURFACE ( 'NONE', #4570, 3.000000000000002665 ) ;
#10682=VECTOR ( 'NONE', #3835, 1000.000000000000000 ) ;
#10695=EDGE_CURVE ( 'NONE', #9455, #8020, #8337, .T. ) ;
#10700=DIRECTION ( 'NONE',  ( 1.000000000000000000, 0.000000000000000000, 0.000000000000000000 ) ) ;
#10745=CARTESIAN_POINT ( 'NONE',  ( 63.44486372867152824, 109.8897274573438096, -15.00000000000000000 ) ) ;
#10769=EDGE_CURVE ( 'NONE', #14522, #11598, #8550, .T. ) ;
#10783=DIRECTION ( 'NONE',  ( 1.000000000000000000, 0.000000000000000000, 0.000000000000000000 ) ) ;
#10792=ORIENTED_EDGE ( 'NONE', *, *, #13563, .T. ) ;
#10856=VECTOR ( 'NONE', #16124, 1000.000000000000000 ) ;
#10871=LINE ( 'NONE', #20181, #10190 ) ;
#10872=DIRECTION ( 'NONE',  ( 1.000000000000000000, 0.000000000000000000, 0.000000000000000000 ) ) ;
#10905=EDGE_CURVE ( 'NONE', #10978, #19490, #3222, .T. ) ;
#10907=ORIENTED_EDGE ( 'NONE', *, *, #20924, .F. ) ;
#10947=DIRECTION ( 'NONE',  ( 1.000000000000000000, 0.000000000000000000, 0.000000000000000000 ) ) ;
#10948=ORIENTED_EDGE ( 'NONE', *, *, #7907, .T. ) ;
#10975=ADVANCED_FACE ( 'NONE', ( #19297, #23745 ), #3150, .F. ) ;
#10978=VERTEX_POINT ( 'NONE', #16860 ) ;
#11012=CARTESIAN_POINT ( 'NONE',  ( 0.000000000000000000, 0.000000000000000000, 18.00000000000000000 ) ) ;
#11026=UNCERTAINTY_MEASURE_WITH_UNIT (LENGTH_MEASURE( 1.000000000000000082E-05 ), #26354, 'distance_accuracy_value', 'NONE');
#11043=ORIENTED_EDGE ( 'NONE', *, *, #30257, .T. ) ;
#11077=DIRECTION ( 'NONE',  ( -0.000000000000000000, 0.000000000000000000, 1.000000000000000000 ) ) ;
#11100=FACE_OUTER_BOUND ( 'NONE', #10032, .T. ) ;
#11138=CIRCLE ( 'NONE', #23839, 3.000000000000002665 ) ;
#11167=CARTESIAN_POINT ( 'NONE',  ( 146.4575131106458912, -10.00000000000001599, -186.4312945166758482 ) ) ;
#11173=CARTESIAN_POINT ( 'NONE',  ( 0.000000000000000000, 0.000000000000000000, 18.00000000000000000 ) ) ;
#11245=EDGE_CURVE ( 'NONE', #930, #4943, #12186, .T. ) ;
#11312=DIRECTION ( 'NONE',  ( 0.000000000000000000, 0.000000000000000000, 1.000000000000000000 ) ) ;
#11367=CARTESIAN_POINT ( 'NONE',  ( 0.000000000000000000, 0.000000000000000000, 18.00000000000000000 ) ) ;
#11381=AXIS2_PLACEMENT_3D ( 'NONE', #9055, #20968, #2378 ) ;
#11465=DIRECTION ( 'NONE',  ( -1.000000000000000000, 0.000000000000000000, 0.000000000000000000 ) ) ;
#11468=EDGE_LOOP ( 'NONE', ( #14925, #13135, #28504, #18878 ) ) ;
#11472=AXIS2_PLACEMENT_3D ( 'NONE', #26335, #28649, #10280 ) ;
#11488=ORIENTED_EDGE ( 'NONE', *, *, #7905, .F. ) ;
#11497=AXIS2_PLACEMENT_3D ( 'NONE', #24991, #2097, #16253 ) ;
#11514=ORIENTED_EDGE ( 'NONE', *, *, #3483, .F. ) ;
#11522=AXIS2_PLACEMENT_3D ( 'NONE', #1745, #13619, #20189 ) ;
#11530=LINE ( 'NONE', #26170, #8393 ) ;
#11533=DIRECTION ( 'NONE',  ( -0.000000000000000000, 0.000000000000000000, 1.000000000000000000 ) ) ;
#11534=EDGE_CURVE ( 'NONE', #23150, #19629, #13504, .T. ) ;
#11537=CIRCLE ( 'NONE', #27204, 3.000000000000002665 ) ;
#11598=VERTEX_POINT ( 'NONE', #14220 ) ;
#11606=ORIENTED_EDGE ( 'NONE', *, *, #30257, .F. ) ;
#11651=EDGE_CURVE ( 'NONE', #20109, #16265, #27695, .T. ) ;
#11665=FILL_AREA_STYLE ('',( #28045 ) ) ;
#11668=CARTESIAN_POINT ( 'NONE',  ( 0.000000000000000000, 0.000000000000000000, 15.00000000000000000 ) ) ;
#11680=VECTOR ( 'NONE', #3758, 1000.000000000000000 ) ;
#11690=CARTESIAN_POINT ( 'NONE',  ( 130.7287565553229456, -4.999999999999983125, 0.5000000000000052180 ) ) ;
#11705=CARTESIAN_POINT ( 'NONE',  ( 172.7287565553229456, -4.999999999999970690, 0.5000000000000029976 ) ) ;
#11728=FACE_BOUND ( 'NONE', #24152, .T. ) ;
#11753=VERTEX_POINT ( 'NONE', #17416 ) ;
#11775=DIRECTION ( 'NONE',  ( 1.000000000000000000, 0.000000000000000000, 0.000000000000000000 ) ) ;
#11794=AXIS2_PLACEMENT_3D ( 'NONE', #14159, #5319, #2446 ) ;
#11803=CARTESIAN_POINT ( 'NONE',  ( 175.7287565553229456, -4.999999999999970690, 3.500000000000003109 ) ) ;
#11807=CARTESIAN_POINT ( 'NONE',  ( 133.7287565553229456, -4.999999999999981348, 0.5000000000000029976 ) ) ;
#11816=VERTEX_POINT ( 'NONE', #22011 ) ;
#11843=ORIENTED_EDGE ( 'NONE', *, *, #18758, .T. ) ;
#11846=DIRECTION ( 'NONE',  ( 0.000000000000000000, 0.000000000000000000, 1.000000000000000000 ) ) ;
#11936=EDGE_LOOP ( 'NONE', ( #7749, #21398, #29369, #17713 ) ) ;
#12014=EDGE_LOOP ( 'NONE', ( #15233, #11043, #9860, #16172 ) ) ;
#12024=AXIS2_PLACEMENT_3D ( 'NONE', #2877, #19485, #721 ) ;
#12068=ORIENTED_EDGE ( 'NONE', *, *, #23765, .F. ) ;
#12082=ORIENTED_EDGE ( 'NONE', *, *, #1936, .T. ) ;
#12110=LINE ( 'NONE', #12405, #6840 ) ;
#12117=EDGE_LOOP ( 'NONE', ( #2728, #14679, #9872, #12082 ) ) ;
#12165=CYLINDRICAL_SURFACE ( 'NONE', #13173, 5.000000000000000000 ) ;
#12186=CIRCLE ( 'NONE', #3428, 139.8897274573438096 ) ;
#12197=AXIS2_PLACEMENT_3D ( 'NONE', #19505, #10193, #3500 ) ;
#12218=CIRCLE ( 'NONE', #8318, 49.99999999999998579 ) ;
#12239=CARTESIAN_POINT ( 'NONE',  ( 120.0000000000000000, 20.00000000000000355, -186.4312945166758482 ) ) ;
#12245=VERTEX_POINT ( 'NONE', #17530 ) ;
#12272=ORIENTED_EDGE ( 'NONE', *, *, #15257, .F. ) ;
#12273=DIRECTION ( 'NONE',  ( -1.000000000000000000, 0.000000000000000000, 0.000000000000000000 ) ) ;
#12319=CARTESIAN_POINT ( 'NONE',  ( -11.85189716074913058, -5.341585316273319783, 4.999999999999998224 ) ) ;
#12334=ORIENTED_EDGE ( 'NONE', *, *, #10309, .F. ) ;
#12385=LINE ( 'NONE', #10091, #15615 ) ;
#12405=CARTESIAN_POINT ( 'NONE',  ( 8.000000000000000000, 9.797174393178825657E-16, 18.00000000000000000 ) ) ;
#12461=CIRCLE ( 'NONE', #26133, 13.00000000000000178 ) ;
#12485=ORIENTED_EDGE ( 'NONE', *, *, #27938, .T. ) ;
#12493=CIRCLE ( 'NONE', #24703, 8.000000000000000000 ) ;
#12557=CARTESIAN_POINT ( 'NONE',  ( 130.7287565553229456, -4.999999999999983125, 3.500000000000003109 ) ) ;
#12639=AXIS2_PLACEMENT_3D ( 'NONE', #4986, #2571, #21466 ) ;
#12655=ORIENTED_EDGE ( 'NONE', *, *, #9834, .T. ) ;
#12659=AXIS2_PLACEMENT_3D ( 'NONE', #3991, #18470, #13290 ) ;
#12665=CIRCLE ( 'NONE', #988, 13.00000000000000178 ) ;
#12674=AXIS2_PLACEMENT_3D ( 'NONE', #12239, #14966, #1117 ) ;
#12688=DIRECTION ( 'NONE',  ( 0.000000000000000000, 0.000000000000000000, 1.000000000000000000 ) ) ;
#12707=EDGE_LOOP ( 'NONE', ( #11514, #23948, #23349, #23767, #249, #20794, #8116, #24455 ) ) ;
#12726=CYLINDRICAL_SURFACE ( 'NONE', #22002, 3.000000000000002665 ) ;
#12770=DIRECTION ( 'NONE',  ( 0.000000000000000000, 0.000000000000000000, 1.000000000000000000 ) ) ;
#12788=CARTESIAN_POINT ( 'NONE',  ( 130.7287565553229456, -4.999999999999983125, 3.500000000000003109 ) ) ;
#12815=CARTESIAN_POINT ( 'NONE',  ( 13.00000000000000178, 0.000000000000000000, 4.999999999999998224 ) ) ;
#12888=SHAPE_REPRESENTATION_RELATIONSHIP ( 'NONE' , 'NONE' ,  #17708, #28104 ) ;
#12892=EDGE_CURVE ( 'NONE', #9080, #20712, #19387, .T. ) ;
#12916=ORIENTED_EDGE ( 'NONE', *, *, #9628, .T. ) ;
#12986=CARTESIAN_POINT ( 'NONE',  ( -20.00000000000017053, 34.64101615137744972, 4.999999999999998224 ) ) ;
#13002=CARTESIAN_POINT ( 'NONE',  ( 175.7287565553229456, -9.999999999999971578, 0.5000000000000029976 ) ) ;
#13034=ORIENTED_EDGE ( 'NONE', *, *, #8865, .F. ) ;
#13076=ORIENTED_EDGE ( 'NONE', *, *, #23166, .T. ) ;
#13079=VECTOR ( 'NONE', #7305, 1000.000000000000000 ) ;
#13084=CARTESIAN_POINT ( 'NONE',  ( 130.7287565553229172, -4.999999999999983125, -36.50000000000000711 ) ) ;
#13134=CARTESIAN_POINT ( 'NONE',  ( 172.7287565553229456, -4.999999999999971578, 3.500000000000003109 ) ) ;
#13135=ORIENTED_EDGE ( 'NONE', *, *, #14057, .F. ) ;
#13148=VERTEX_POINT ( 'NONE', #23357 ) ;
#13153=ORIENTED_EDGE ( 'NONE', *, *, #4435, .T. ) ;
#13173=AXIS2_PLACEMENT_3D ( 'NONE', #7145, #9719, #7450 ) ;
#13190=AXIS2_PLACEMENT_3D ( 'NONE', #5435, #19606, #10446 ) ;
#13210=CARTESIAN_POINT ( 'NONE',  ( 0.000000000000000000, 0.000000000000000000, -15.00000000000000355 ) ) ;
#13224=ADVANCED_FACE ( 'NONE', ( #7036 ), #20340, .T. ) ;
#13268=ORIENTED_EDGE ( 'NONE', *, *, #5551, .F. ) ;
#13290=DIRECTION ( 'NONE',  ( 0.4108911781748707526, -0.9116843969807022496, 0.000000000000000000 ) ) ;
#13302=CARTESIAN_POINT ( 'NONE',  ( -11.85189716074912880, -5.341585316273318895, 9.999999999999998224 ) ) ;
#13329=ORIENTED_EDGE ( 'NONE', *, *, #10769, .F. ) ;
#13371=PLANE ( 'NONE',  #4668 ) ;
#13441=VERTEX_POINT ( 'NONE', #9906 ) ;
#13448=EDGE_CURVE ( 'NONE', #24792, #6067, #14040, .T. ) ;
#13478=ADVANCED_FACE ( 'NONE', ( #23979 ), #10054, .T. ) ;
#13504=CIRCLE ( 'NONE', #26699, 8.000000000000000000 ) ;
#13536=VECTOR ( 'NONE', #16196, 1000.000000000000000 ) ;
#13553=ORIENTED_EDGE ( 'NONE', *, *, #10905, .F. ) ;
#13563=EDGE_CURVE ( 'NONE', #20421, #3893, #20124, .T. ) ;
#13609=CARTESIAN_POINT ( 'NONE',  ( 160.0000000000000000, -10.00000000000000000, -15.00000000000000000 ) ) ;
#13618=ORIENTED_EDGE ( 'NONE', *, *, #25069, .T. ) ;
#13619=DIRECTION ( 'NONE',  ( 2.698458740408365879E-16, -1.000000000000000000, 0.000000000000000000 ) ) ;
#13663=DIRECTION ( 'NONE',  ( 1.000000000000000000, 0.000000000000000000, 0.000000000000000000 ) ) ;
#13781=ORIENTED_EDGE ( 'NONE', *, *, #28910, .T. ) ;
#13800=FACE_OUTER_BOUND ( 'NONE', #3661, .T. ) ;
#13862=EDGE_LOOP ( 'NONE', ( #10948, #18732, #27604, #13618, #13781, #8417, #23421, #30031 ) ) ;
#13903=AXIS2_PLACEMENT_3D ( 'NONE', #7103, #26190, #395 ) ;
#13947=SURFACE_STYLE_FILL_AREA ( #11665 ) ;
#13953=ORIENTED_EDGE ( 'NONE', *, *, #14540, .T. ) ;
#14015=AXIS2_PLACEMENT_3D ( 'NONE', #25513, #15884, #27540 ) ;
#14024=LINE ( 'NONE', #465, #1467 ) ;
#14040=CIRCLE ( 'NONE', #24298, 4.000000000000000000 ) ;
#14051=DIRECTION ( 'NONE',  ( 0.000000000000000000, 0.000000000000000000, 1.000000000000000000 ) ) ;
#14057=EDGE_CURVE ( 'NONE', #3119, #15024, #21627, .T. ) ;
#14088=AXIS2_PLACEMENT_3D ( 'NONE', #1176, #26830, #22072 ) ;
#14149=DIRECTION ( 'NONE',  ( 1.000000000000000000, 0.000000000000000000, 0.000000000000000000 ) ) ;
#14159=CARTESIAN_POINT ( 'NONE',  ( 172.7287565553229456, -4.999999999999971578, 0.5000000000000029976 ) ) ;
#14162=VECTOR ( 'NONE', #5757, 1000.000000000000000 ) ;
#14197=DIRECTION ( 'NONE',  ( 1.000000000000000000, 0.000000000000000000, 0.000000000000000000 ) ) ;
#14206=ORIENTED_EDGE ( 'NONE', *, *, #3604, .F. ) ;
#14212=DIRECTION ( 'NONE',  ( 1.000000000000000000, 1.280948979423041604E-16, -0.000000000000000000 ) ) ;
#14220=CARTESIAN_POINT ( 'NONE',  ( -24.00000000000017053, 34.64101615137744972, 9.999999999999998224 ) ) ;
#14235=ADVANCED_FACE ( 'NONE', ( #8344 ), #13371, .F. ) ;
#14252=LINE ( 'NONE', #9833, #1505 ) ;
#14283=EDGE_LOOP ( 'NONE', ( #19426, #3230, #20558, #22734 ) ) ;
#14289=EDGE_LOOP ( 'NONE', ( #27883, #14927, #24595, #4582 ) ) ;
#14318=VERTEX_POINT ( 'NONE', #7109 ) ;
#14327=CARTESIAN_POINT ( 'NONE',  ( 0.000000000000000000, 0.000000000000000000, -15.00000000000000000 ) ) ;
#14333=ORIENTED_EDGE ( 'NONE', *, *, #15334, .F. ) ;
#14339=ORIENTED_EDGE ( 'NONE', *, *, #21790, .T. ) ;
#14384=EDGE_LOOP ( 'NONE', ( #4749, #8832, #7979, #14206 ) ) ;
#14415=VERTEX_POINT ( 'NONE', #18709 ) ;
#14522=VERTEX_POINT ( 'NONE', #10139 ) ;
#14523=CARTESIAN_POINT ( 'NONE',  ( 130.7287565553229172, -4.999999999999983125, -33.50000000000000000 ) ) ;
#14540=EDGE_CURVE ( 'NONE', #1338, #24750, #26347, .T. ) ;
#14562=CARTESIAN_POINT ( 'NONE',  ( -13.00000000000000178, 0.000000000000000000, -15.00000000000000000 ) ) ;
#14632=DIRECTION ( 'NONE',  ( 1.000000000000000000, 0.000000000000000000, 0.000000000000000000 ) ) ;
#14679=ORIENTED_EDGE ( 'NONE', *, *, #28100, .T. ) ;
#14694=DIRECTION ( 'NONE',  ( 0.000000000000000000, 0.000000000000000000, -1.000000000000000000 ) ) ;
#14707=VECTOR ( 'NONE', #11312, 1000.000000000000000 ) ;
#14721=AXIS2_PLACEMENT_3D ( 'NONE', #11173, #6304, #24931 ) ;
#14925=ORIENTED_EDGE ( 'NONE', *, *, #26222, .F. ) ;
#14927=ORIENTED_EDGE ( 'NONE', *, *, #17365, .F. ) ;
#14958=DIRECTION ( 'NONE',  ( 0.000000000000000000, 0.000000000000000000, 1.000000000000000000 ) ) ;
#14966=DIRECTION ( 'NONE',  ( 0.000000000000000000, 0.000000000000000000, 1.000000000000000000 ) ) ;
#14977=DIRECTION ( 'NONE',  ( 0.000000000000000000, 0.000000000000000000, -1.000000000000000000 ) ) ;
#15024=VERTEX_POINT ( 'NONE', #15924 ) ;
#15091=PRODUCT_DEFINITION ( 'UNKNOWN', '', #27823, #15569 ) ;
#15104=AXIS2_PLACEMENT_3D ( 'NONE', #29576, #15618, #8593 ) ;
#15110=CARTESIAN_POINT ( 'NONE',  ( 13.00000000000000178, 1.592040838891559293E-15, -15.00000000000000000 ) ) ;
#15135=DIRECTION ( 'NONE',  ( -0.000000000000000000, 0.000000000000000000, 1.000000000000000000 ) ) ;
#15143=AXIS2_PLACEMENT_3D ( 'NONE', #27748, #16559, #18845 ) ;
#15154=FACE_OUTER_BOUND ( 'NONE', #25326, .T. ) ;
#15160=VERTEX_POINT ( 'NONE', #2976 ) ;
#15182=CARTESIAN_POINT ( 'NONE',  ( 0.000000000000000000, 0.000000000000000000, -18.00000000000000000 ) ) ;
#15199=DIRECTION ( 'NONE',  ( 2.908569913943825554E-16, -1.000000000000000000, 0.000000000000000000 ) ) ;
#15206=EDGE_CURVE ( 'NONE', #25233, #25802, #19421, .T. ) ;
#15220=FACE_BOUND ( 'NONE', #26144, .T. ) ;
#15233=ORIENTED_EDGE ( 'NONE', *, *, #21384, .T. ) ;
#15249=DIRECTION ( 'NONE',  ( 2.698458740408365879E-16, -1.000000000000000000, 0.000000000000000000 ) ) ;
#15257=EDGE_CURVE ( 'NONE', #2706, #29352, #21261, .T. ) ;
#15331=EDGE_CURVE ( 'NONE', #29853, #4723, #1274, .T. ) ;
#15334=EDGE_CURVE ( 'NONE', #19629, #23150, #12493, .T. ) ;
#15346=CARTESIAN_POINT ( 'NONE',  ( 8.000000000000000000, 9.797174393178825657E-16, 9.999999999999998224 ) ) ;
#15373=DIRECTION ( 'NONE',  ( 0.000000000000000000, 0.000000000000000000, -1.000000000000000000 ) ) ;
#15376=EDGE_CURVE ( 'NONE', #9938, #19084, #16402, .T. ) ;
#15426=CIRCLE ( 'NONE', #2297, 13.00000000000000178 ) ;
#15529=DIRECTION ( 'NONE',  ( -1.000000000000000000, 0.000000000000000000, 0.000000000000000000 ) ) ;
#15531=( NAMED_UNIT ( * ) SI_UNIT ( $, .STERADIAN. ) SOLID_ANGLE_UNIT ( ) );
#15555=ADVANCED_FACE ( 'NONE', ( #8717 ), #6450, .F. ) ;
#15569=PRODUCT_DEFINITION_CONTEXT ( 'detailed design', #18251, 'design' ) ;
#15588=EDGE_CURVE ( 'NONE', #17672, #20109, #20315, .T. ) ;
#15604=DIRECTION ( 'NONE',  ( -2.908569913943825554E-16, 1.000000000000000000, -0.000000000000000000 ) ) ;
#15609=DIRECTION ( 'NONE',  ( 0.000000000000000000, 0.000000000000000000, -1.000000000000000000 ) ) ;
#15615=VECTOR ( 'NONE', #12688, 1000.000000000000000 ) ;
#15618=DIRECTION ( 'NONE',  ( 0.000000000000000000, 0.000000000000000000, 1.000000000000000000 ) ) ;
#15642=ORIENTED_EDGE ( 'NONE', *, *, #2676, .F. ) ;
#15674=EDGE_LOOP ( 'NONE', ( #26648, #13953, #25963, #5056 ) ) ;
#15684=EDGE_CURVE ( 'NONE', #2471, #24619, #15697, .T. ) ;
#15697=CIRCLE ( 'NONE', #22047, 13.00000000000000178 ) ;
#15720=ORIENTED_EDGE ( 'NONE', *, *, #21269, .T. ) ;
#15884=DIRECTION ( 'NONE',  ( 0.000000000000000000, 0.000000000000000000, 1.000000000000000000 ) ) ;
#15924=CARTESIAN_POINT ( 'NONE',  ( -28.20515957282649921, 30.94299554780361206, 9.999999999999998224 ) ) ;
#15975=PLANE ( 'NONE',  #27961 ) ;
#15976=DIRECTION ( 'NONE',  ( 0.000000000000000000, 0.000000000000000000, 1.000000000000000000 ) ) ;
#15998=ORIENTED_EDGE ( 'NONE', *, *, #1318, .F. ) ;
#16052=AXIS2_PLACEMENT_3D ( 'NONE', #6837, #6236, #15529 ) ;
#16056=EDGE_LOOP ( 'NONE', ( #257, #6822 ) ) ;
#16077=VERTEX_POINT ( 'NONE', #18454 ) ;
#16112=APPLICATION_CONTEXT ( 'automotive_design' ) ;
#16124=DIRECTION ( 'NONE',  ( -2.908569913943825554E-16, 1.000000000000000000, -0.000000000000000000 ) ) ;
#16130=VECTOR ( 'NONE', #5452, 1000.000000000000000 ) ;
#16136=ADVANCED_FACE ( 'NONE', ( #7604 ), #16909, .T. ) ;
#16165=AXIS2_PLACEMENT_3D ( 'NONE', #19427, #26023, #23570 ) ;
#16172=ORIENTED_EDGE ( 'NONE', *, *, #20371, .F. ) ;
#16180=ORIENTED_EDGE ( 'NONE', *, *, #995, .T. ) ;
#16196=DIRECTION ( 'NONE',  ( 0.4108911781748706971, -0.9116843969807022496, 0.000000000000000000 ) ) ;
#16206=DIRECTION ( 'NONE',  ( 0.000000000000000000, 0.000000000000000000, 1.000000000000000000 ) ) ;
#16209=CYLINDRICAL_SURFACE ( 'NONE', #5111, 3.000000000000002665 ) ;
#16211=CARTESIAN_POINT ( 'NONE',  ( -8.000000000000000000, 0.000000000000000000, 15.00000000000000000 ) ) ;
#16247=( NAMED_UNIT ( * ) PLANE_ANGLE_UNIT ( ) SI_UNIT ( $, .RADIAN. ) );
#16253=DIRECTION ( 'NONE',  ( 1.000000000000000000, 0.000000000000000000, 0.000000000000000000 ) ) ;
#16265=VERTEX_POINT ( 'NONE', #27954 ) ;
#16272=DIRECTION ( 'NONE',  ( 0.000000000000000000, 0.000000000000000000, -1.000000000000000000 ) ) ;
#16275=CARTESIAN_POINT ( 'NONE',  ( 8.000000000000000000, 9.797174393178825657E-16, 15.00000000000000000 ) ) ;
#16304=EDGE_CURVE ( 'NONE', #24792, #11598, #19346, .T. ) ;
#16367=CARTESIAN_POINT ( 'NONE',  ( 120.0000000000000000, 20.00000000000000355, -15.00000000000000000 ) ) ;
#16402=CIRCLE ( 'NONE', #16883, 8.000000000000000000 ) ;
#16426=AXIS2_PLACEMENT_3D ( 'NONE', #16367, #9647, #4776 ) ;
#16437=CARTESIAN_POINT ( 'NONE',  ( 130.7287565553229456, -9.999999999999982236, 3.500000000000003109 ) ) ;
#16440=FACE_BOUND ( 'NONE', #21845, .T. ) ;
#16449=DIRECTION ( 'NONE',  ( 0.000000000000000000, 0.000000000000000000, 1.000000000000000000 ) ) ;
#16452=CIRCLE ( 'NONE', #21815, 13.00000000000000178 ) ;
#16460=CARTESIAN_POINT ( 'NONE',  ( 0.000000000000000000, 0.000000000000000000, -18.00000000000000000 ) ) ;
#16506=DIRECTION ( 'NONE',  ( -0.000000000000000000, -0.000000000000000000, -1.000000000000000000 ) ) ;
#16551=CARTESIAN_POINT ( 'NONE',  ( 120.0000000000000000, -19.99999999999999645, -17.99999999999998934 ) ) ;
#16559=DIRECTION ( 'NONE',  ( 0.000000000000000000, 0.000000000000000000, 1.000000000000000000 ) ) ;
#16571=ORIENTED_EDGE ( 'NONE', *, *, #15334, .T. ) ;
#16605=ORIENTED_EDGE ( 'NONE', *, *, #20276, .T. ) ;
#16616=DIRECTION ( 'NONE',  ( 1.000000000000000000, 0.000000000000000000, 0.000000000000000000 ) ) ;
#16660=ADVANCED_FACE ( 'NONE', ( #3791 ), #20248, .F. ) ;
#16678=ORIENTED_EDGE ( 'NONE', *, *, #23597, .T. ) ;
#16681=ORIENTED_EDGE ( 'NONE', *, *, #5500, .F. ) ;
#16688=EDGE_LOOP ( 'NONE', ( #15998, #16180, #17158, #23564 ) ) ;
#16694=ORIENTED_EDGE ( 'NONE', *, *, #1552, .T. ) ;
#16698=AXIS2_PLACEMENT_3D ( 'NONE', #9737, #2743, #16616 ) ;
#16764=CARTESIAN_POINT ( 'NONE',  ( 0.000000000000000000, 0.000000000000000000, -15.00000000000000355 ) ) ;
#16790=ORIENTED_EDGE ( 'NONE', *, *, #1581, .T. ) ;
#16793=VERTEX_POINT ( 'NONE', #7538 ) ;
#16810=CARTESIAN_POINT ( 'NONE',  ( 63.44486372867149981, -20.00000000000000355, -17.99999999999998934 ) ) ;
#16826=EDGE_CURVE ( 'NONE', #28576, #17347, #11530, .T. ) ;
#16835=ORIENTED_EDGE ( 'NONE', *, *, #26597, .F. ) ;
#16851=VECTOR ( 'NONE', #7553, 1000.000000000000000 ) ;
#16860=CARTESIAN_POINT ( 'NONE',  ( -13.00000000000000178, 1.592040838891559293E-15, 15.00000000000000000 ) ) ;
#16875=CIRCLE ( 'NONE', #17342, 139.8897274573438096 ) ;
#16879=ORIENTED_EDGE ( 'NONE', *, *, #7407, .T. ) ;
#16883=AXIS2_PLACEMENT_3D ( 'NONE', #17285, #10565, #10258 ) ;
#16909=CYLINDRICAL_SURFACE ( 'NONE', #11794, 3.000000000000002665 ) ;
#16955=DIRECTION ( 'NONE',  ( 0.000000000000000000, 0.000000000000000000, -1.000000000000000000 ) ) ;
#17002=DIRECTION ( 'NONE',  ( -2.698458740408365879E-16, 1.000000000000000000, -0.000000000000000000 ) ) ;
#17036=DIRECTION ( 'NONE',  ( 0.000000000000000000, 0.000000000000000000, -1.000000000000000000 ) ) ;
#17099=LINE ( 'NONE', #10220, #23318 ) ;
#17146=EDGE_LOOP ( 'NONE', ( #30017, #28525 ) ) ;
#17158=ORIENTED_EDGE ( 'NONE', *, *, #10382, .T. ) ;
#17163=FACE_OUTER_BOUND ( 'NONE', #7239, .T. ) ;
#17167=DIRECTION ( 'NONE',  ( 0.000000000000000000, 0.000000000000000000, 1.000000000000000000 ) ) ;
#17224=VECTOR ( 'NONE', #8167, 1000.000000000000000 ) ;
#17247=ORIENTED_EDGE ( 'NONE', *, *, #9834, .F. ) ;
#17285=CARTESIAN_POINT ( 'NONE',  ( 0.000000000000000000, 0.000000000000000000, 15.00000000000000000 ) ) ;
#17336=CARTESIAN_POINT ( 'NONE',  ( 63.44486372867152824, -29.99999999999998934, -17.99999999999998934 ) ) ;
#17342=AXIS2_PLACEMENT_3D ( 'NONE', #29772, #17937, #30062 ) ;
#17347=VERTEX_POINT ( 'NONE', #7280 ) ;
#17363=CARTESIAN_POINT ( 'NONE',  ( 10.55189716074911921, 7.593251366112848899, 4.999999999999998224 ) ) ;
#17365=EDGE_CURVE ( 'NONE', #25802, #19921, #25748, .T. ) ;
#17372=ADVANCED_FACE ( 'NONE', ( #27921, #8945, #18262 ), #15975, .T. ) ;
#17401=LINE ( 'NONE', #10533, #10682 ) ;
#17416=CARTESIAN_POINT ( 'NONE',  ( 10.55189716074911921, 7.593251366112849787, 9.999999999999998224 ) ) ;
#17481=EDGE_CURVE ( 'NONE', #4723, #27841, #22089, .T. ) ;
#17512=VERTEX_POINT ( 'NONE', #867 ) ;
#17514=DIRECTION ( 'NONE',  ( 1.000000000000000000, 0.000000000000000000, 0.000000000000000000 ) ) ;
#17530=CARTESIAN_POINT ( 'NONE',  ( 160.0000000000000284, -9.999999999999973355, -17.99999999999998934 ) ) ;
#17623=ORIENTED_EDGE ( 'NONE', *, *, #11245, .T. ) ;
#17658=AXIS2_PLACEMENT_3D ( 'NONE', #13084, #24853, #1511 ) ;
#17672=VERTEX_POINT ( 'NONE', #19760 ) ;
#17707=EDGE_CURVE ( 'NONE', #30082, #22823, #6042, .T. ) ;
#17708=SHAPE_REPRESENTATION ( 'pedal', ( #13190 ), #24415 ) ;
#17710=ORIENTED_EDGE ( 'NONE', *, *, #23765, .T. ) ;
#17713=ORIENTED_EDGE ( 'NONE', *, *, #9583, .F. ) ;
#17723=ORIENTED_EDGE ( 'NONE', *, *, #15376, .F. ) ;
#17818=EDGE_CURVE ( 'NONE', #10508, #17512, #7958, .T. ) ;
#17827=ORIENTED_EDGE ( 'NONE', *, *, #28100, .F. ) ;
#17848=DIRECTION ( 'NONE',  ( -6.938893903907227392E-16, 0.000000000000000000, -1.000000000000000000 ) ) ;
#17856=CARTESIAN_POINT ( 'NONE',  ( 13.00000000000000178, 1.592040838891559293E-15, -18.00000000000000000 ) ) ;
#17874=FACE_OUTER_BOUND ( 'NONE', #28376, .T. ) ;
#17881=CARTESIAN_POINT ( 'NONE',  ( 0.000000000000000000, 0.000000000000000000, 15.00000000000000000 ) ) ;
#17901=PLANE ( 'NONE',  #23465 ) ;
#17933=DIRECTION ( 'NONE',  ( 1.000000000000000000, 0.000000000000000000, 0.000000000000000000 ) ) ;
#17937=DIRECTION ( 'NONE',  ( -0.000000000000000000, -0.000000000000000000, -1.000000000000000000 ) ) ;
#17961=CYLINDRICAL_SURFACE ( 'NONE', #16052, 8.000000000000000000 ) ;
#17994=ADVANCED_FACE ( 'NONE', ( #19281 ), #26325, .F. ) ;
#18060=ORIENTED_EDGE ( 'NONE', *, *, #13563, .F. ) ;
#18066=DIRECTION ( 'NONE',  ( 1.000000000000000000, 0.000000000000000000, 0.000000000000000000 ) ) ;
#18116=( LENGTH_UNIT ( ) NAMED_UNIT ( * ) SI_UNIT ( .MILLI., .METRE. ) );
#18147=CARTESIAN_POINT ( 'NONE',  ( -11.85189716074913058, -5.341585316273319783, 4.999999999999998224 ) ) ;
#18155=ORIENTED_EDGE ( 'NONE', *, *, #25376, .F. ) ;
#18189=CIRCLE ( 'NONE', #669, 13.00000000000000178 ) ;
#18193=DIRECTION ( 'NONE',  ( 1.000000000000000000, 2.891205793294675861E-16, 0.000000000000000000 ) ) ;
#18251=APPLICATION_CONTEXT ( 'automotive_design' ) ;
#18262=FACE_BOUND ( 'NONE', #28079, .T. ) ;
#18282=ORIENTED_EDGE ( 'NONE', *, *, #13448, .T. ) ;
#18334=ORIENTED_EDGE ( 'NONE', *, *, #1936, .F. ) ;
#18341=ORIENTED_EDGE ( 'NONE', *, *, #5551, .T. ) ;
#18374=AXIS2_PLACEMENT_3D ( 'NONE', #12986, #1406, #10700 ) ;
#18433=CARTESIAN_POINT ( 'NONE',  ( 34.54859390953723874, -22.18451583373416014, -15.00000000000000000 ) ) ;
#18444=DIRECTION ( 'NONE',  ( 1.000000000000000000, 0.000000000000000000, 0.000000000000000000 ) ) ;
#18454=CARTESIAN_POINT ( 'NONE',  ( 13.00000000000000178, 0.000000000000000000, 9.999999999999998224 ) ) ;
#18470=DIRECTION ( 'NONE',  ( -0.9116843969807022496, -0.4108911781748707526, 0.000000000000000000 ) ) ;
#18504=EDGE_LOOP ( 'NONE', ( #16879, #8944, #4742, #16605 ) ) ;
#18537=AXIS2_PLACEMENT_3D ( 'NONE', #24300, #7960, #25998 ) ;
#18544=( LENGTH_UNIT ( ) NAMED_UNIT ( * ) SI_UNIT ( .MILLI., .METRE. ) );
#18625=EDGE_LOOP ( 'NONE', ( #26917, #20680, #8190, #29819 ) ) ;
#18629=DIRECTION ( 'NONE',  ( -1.000000000000000000, 0.000000000000000000, 0.000000000000000000 ) ) ;
#18643=PLANE ( 'NONE',  #24265 ) ;
#18653=ADVANCED_FACE ( 'NONE', ( #26246 ), #742, .F. ) ;
#18655=LINE ( 'NONE', #28000, #28262 ) ;
#18661=DIRECTION ( 'NONE',  ( 1.000000000000000000, 0.000000000000000000, 0.000000000000000000 ) ) ;
#18682=ORIENTED_EDGE ( 'NONE', *, *, #25376, .T. ) ;
#18709=CARTESIAN_POINT ( 'NONE',  ( 130.7287565553229172, -4.999999999999983125, -33.50000000000000000 ) ) ;
#18732=ORIENTED_EDGE ( 'NONE', *, *, #21516, .T. ) ;
#18734=CARTESIAN_POINT ( 'NONE',  ( 63.44486372867149981, -20.00000000000003197, -15.00000000000000000 ) ) ;
#18737=DIRECTION ( 'NONE',  ( 1.000000000000000000, 0.000000000000000000, 0.000000000000000000 ) ) ;
#18748=CARTESIAN_POINT ( 'NONE',  ( 146.4575131106458912, -10.00000000000000178, -15.00000000000000000 ) ) ;
#18750=AXIS2_PLACEMENT_3D ( 'NONE', #17881, #22639, #10872 ) ;
#18758=EDGE_CURVE ( 'NONE', #8805, #24538, #26045, .T. ) ;
#18797=ADVANCED_FACE ( 'NONE', ( #3643 ), #10651, .T. ) ;
#18814=LINE ( 'NONE', #14523, #7635 ) ;
#18822=CARTESIAN_POINT ( 'NONE',  ( 9.884967449281287344, -8.443187699361503817, -16.50000000000001421 ) ) ;
#18823=EDGE_CURVE ( 'NONE', #25891, #17512, #4246, .T. ) ;
#18845=DIRECTION ( 'NONE',  ( 1.000000000000000000, 0.000000000000000000, 0.000000000000000000 ) ) ;
#18878=ORIENTED_EDGE ( 'NONE', *, *, #26856, .T. ) ;
#18900=DIRECTION ( 'NONE',  ( -1.000000000000000000, -1.280948979423041851E-16, -0.000000000000000000 ) ) ;
#18932=DIRECTION ( 'NONE',  ( 2.698458740408365879E-16, -1.000000000000000000, 0.000000000000000000 ) ) ;
#18955=DIRECTION ( 'NONE',  ( -0.000000000000000000, -0.000000000000000000, -1.000000000000000000 ) ) ;
#19045=CARTESIAN_POINT ( 'NONE',  ( 130.7287565553229172, -9.999999999999982236, -33.50000000000000000 ) ) ;
#19084=VERTEX_POINT ( 'NONE', #16275 ) ;
#19111=EDGE_LOOP ( 'NONE', ( #18060, #12655, #12272, #13268 ) ) ;
#19166=ORIENTED_EDGE ( 'NONE', *, *, #9869, .T. ) ;
#19170=DIRECTION ( 'NONE',  ( 0.000000000000000000, 0.000000000000000000, 1.000000000000000000 ) ) ;
#19171=CARTESIAN_POINT ( 'NONE',  ( 120.0000000000000000, 20.00000000000000355, -17.99999999999998934 ) ) ;
#19182=CARTESIAN_POINT ( 'NONE',  ( 133.7287565553229456, -4.999999999999982236, 3.500000000000003109 ) ) ;
#19221=CARTESIAN_POINT ( 'NONE',  ( -13.00000000000000178, 0.000000000000000000, -18.00000000000000000 ) ) ;
#19281=FACE_OUTER_BOUND ( 'NONE', #16688, .T. ) ;
#19297=FACE_BOUND ( 'NONE', #7392, .T. ) ;
#19337=EDGE_LOOP ( 'NONE', ( #23970, #4906, #16681, #27062 ) ) ;
#19346=LINE ( 'NONE', #3492, #4506 ) ;
#19352=FACE_OUTER_BOUND ( 'NONE', #16056, .T. ) ;
#19387=CIRCLE ( 'NONE', #10123, 8.000000000000000000 ) ;
#19421=LINE ( 'NONE', #5397, #27169 ) ;
#19426=ORIENTED_EDGE ( 'NONE', *, *, #26828, .F. ) ;
#19427=CARTESIAN_POINT ( 'NONE',  ( 63.44486372867152824, 109.8897274573438096, -15.00000000000000000 ) ) ;
#19466=DIRECTION ( 'NONE',  ( 1.000000000000000000, 0.000000000000000000, 0.000000000000000000 ) ) ;
#19485=DIRECTION ( 'NONE',  ( 0.000000000000000000, 0.000000000000000000, -1.000000000000000000 ) ) ;
#19487=DIRECTION ( 'NONE',  ( 0.000000000000000000, 0.000000000000000000, 1.000000000000000000 ) ) ;
#19490=VERTEX_POINT ( 'NONE', #2383 ) ;
#19500=AXIS2_PLACEMENT_3D ( 'NONE', #454, #28110, #21348 ) ;
#19505=CARTESIAN_POINT ( 'NONE',  ( 0.000000000000000000, 0.000000000000000000, 18.00000000000000000 ) ) ;
#19536=SHAPE_DEFINITION_REPRESENTATION ( #4251, #17708 ) ;
#19547=PLANE ( 'NONE',  #21199 ) ;
#19590=LINE ( 'NONE', #24487, #25316 ) ;
#19606=DIRECTION ( 'NONE',  ( 0.000000000000000000, 0.000000000000000000, 1.000000000000000000 ) ) ;
#19621=DIRECTION ( 'NONE',  ( -0.000000000000000000, 0.000000000000000000, 1.000000000000000000 ) ) ;
#19629=VERTEX_POINT ( 'NONE', #2540 ) ;
#19672=VERTEX_POINT ( 'NONE', #3286 ) ;
#19699=DIRECTION ( 'NONE',  ( -1.000000000000000000, 0.000000000000000000, 0.000000000000000000 ) ) ;
#19729=CARTESIAN_POINT ( 'NONE',  ( 130.7287565553229456, -4.999999999999983125, 0.5000000000000052180 ) ) ;
#19760=CARTESIAN_POINT ( 'NONE',  ( 146.4575131106459196, -9.999999999999976907, -17.99999999999998934 ) ) ;
#19761=EDGE_LOOP ( 'NONE', ( #9084, #19898, #19795, #6839 ) ) ;
#19795=ORIENTED_EDGE ( 'NONE', *, *, #8865, .T. ) ;
#19867=CARTESIAN_POINT ( 'NONE',  ( 0.000000000000000000, 0.000000000000000000, -15.00000000000000000 ) ) ;
#19884=AXIS2_PLACEMENT_3D ( 'NONE', #6321, #28281, #18629 ) ;
#19898=ORIENTED_EDGE ( 'NONE', *, *, #16304, .T. ) ;
#19901=DIRECTION ( 'NONE',  ( -0.000000000000000000, -0.000000000000000000, -1.000000000000000000 ) ) ;
#19914=SURFACE_STYLE_FILL_AREA ( #24653 ) ;
#19921=VERTEX_POINT ( 'NONE', #19729 ) ;
#20000=ADVANCED_FACE ( 'NONE', ( #24783 ), #24477, .T. ) ;
#20012=EDGE_LOOP ( 'NONE', ( #12485, #29332, #20570, #22654, #20848 ) ) ;
#20032=DIRECTION ( 'NONE',  ( 1.000000000000000000, 0.000000000000000000, 0.000000000000000000 ) ) ;
#20039=CIRCLE ( 'NONE', #15143, 1.500000000000001332 ) ;
#20075=CARTESIAN_POINT ( 'NONE',  ( 172.7287565553229456, -4.999999999999970690, 3.500000000000003109 ) ) ;
#20084=CARTESIAN_POINT ( 'NONE',  ( 0.000000000000000000, 0.000000000000000000, 4.999999999999998224 ) ) ;
#20109=VERTEX_POINT ( 'NONE', #2193 ) ;
#20124=LINE ( 'NONE', #10505, #29595 ) ;
#20151=ORIENTED_EDGE ( 'NONE', *, *, #22362, .T. ) ;
#20168=LINE ( 'NONE', #13302, #13536 ) ;
#20181=CARTESIAN_POINT ( 'NONE',  ( -8.000000000000000000, 0.000000000000000000, 18.00000000000000000 ) ) ;
#20189=DIRECTION ( 'NONE',  ( 1.000000000000000000, 2.698458740408365879E-16, 0.000000000000000000 ) ) ;
#20193=CYLINDRICAL_SURFACE ( 'NONE', #15104, 40.00000000000000711 ) ;
#20204=ADVANCED_FACE ( 'NONE', ( #20631 ), #16209, .T. ) ;
#20229=CARTESIAN_POINT ( 'NONE',  ( 119.9999999999999858, -30.00000000000000000, -186.4312945166758482 ) ) ;
#20248=PLANE ( 'NONE',  #17658 ) ;
#20250=EDGE_LOOP ( 'NONE', ( #17710, #4169, #21315, #25895 ) ) ;
#20260=ORIENTED_EDGE ( 'NONE', *, *, #10905, .T. ) ;
#20274=CARTESIAN_POINT ( 'NONE',  ( 133.7287565553229172, -4.999999999999981348, -33.50000000000000000 ) ) ;
#20276=EDGE_CURVE ( 'NONE', #29492, #13148, #5375, .T. ) ;
#20315=LINE ( 'NONE', #11167, #14707 ) ;
#20335=DIRECTION ( 'NONE',  ( -2.698458740408365879E-16, 1.000000000000000000, -0.000000000000000000 ) ) ;
#20340=CYLINDRICAL_SURFACE ( 'NONE', #19884, 8.000000000000000000 ) ;
#20350=FACE_BOUND ( 'NONE', #22793, .T. ) ;
#20371=EDGE_CURVE ( 'NONE', #16793, #24538, #28458, .T. ) ;
#20381=ORIENTED_EDGE ( 'NONE', *, *, #21384, .F. ) ;
#20402=FACE_OUTER_BOUND ( 'NONE', #19761, .T. ) ;
#20421=VERTEX_POINT ( 'NONE', #15110 ) ;
#20470=DIRECTION ( 'NONE',  ( 0.000000000000000000, 0.000000000000000000, 1.000000000000000000 ) ) ;
#20545=ADVANCED_FACE ( 'NONE', ( #6276 ), #19547, .F. ) ;
#20556=DIRECTION ( 'NONE',  ( 1.000000000000000000, 0.000000000000000000, 0.000000000000000000 ) ) ;
#20558=ORIENTED_EDGE ( 'NONE', *, *, #22803, .T. ) ;
#20570=ORIENTED_EDGE ( 'NONE', *, *, #9718, .F. ) ;
#20576=DIRECTION ( 'NONE',  ( -2.698458740408365879E-16, 1.000000000000000000, -0.000000000000000000 ) ) ;
#20615=EDGE_CURVE ( 'NONE', #26545, #16077, #5674, .T. ) ;
#20631=FACE_OUTER_BOUND ( 'NONE', #14289, .T. ) ;
#20632=AXIS2_PLACEMENT_3D ( 'NONE', #12557, #14694, #677 ) ;
#20635=FACE_BOUND ( 'NONE', #14384, .T. ) ;
#20663=DIRECTION ( 'NONE',  ( -1.000000000000000000, 0.000000000000000000, 0.000000000000000000 ) ) ;
#20680=ORIENTED_EDGE ( 'NONE', *, *, #3604, .T. ) ;
#20712=VERTEX_POINT ( 'NONE', #2312 ) ;
#20737=CARTESIAN_POINT ( 'NONE',  ( 133.7287565553229172, -9.999999999999982236, -36.50000000000000711 ) ) ;
#20739=ORIENTED_EDGE ( 'NONE', *, *, #24061, .F. ) ;
#20755=DIRECTION ( 'NONE',  ( 1.000000000000000000, 0.000000000000000000, 0.000000000000000000 ) ) ;
#20794=ORIENTED_EDGE ( 'NONE', *, *, #26560, .T. ) ;
#20848=ORIENTED_EDGE ( 'NONE', *, *, #22803, .F. ) ;
#20851=FACE_OUTER_BOUND ( 'NONE', #25430, .T. ) ;
#20852=ORIENTED_EDGE ( 'NONE', *, *, #26284, .F. ) ;
#20858=ORIENTED_EDGE ( 'NONE', *, *, #16826, .T. ) ;
#20910=CARTESIAN_POINT ( 'NONE',  ( -13.00000000000000178, 1.592040838891559293E-15, 18.00000000000000000 ) ) ;
#20924=EDGE_CURVE ( 'NONE', #10096, #10263, #21650, .T. ) ;
#20968=DIRECTION ( 'NONE',  ( 2.698458740408365879E-16, -1.000000000000000000, 0.000000000000000000 ) ) ;
#21008=CARTESIAN_POINT ( 'NONE',  ( 0.000000000000000000, 0.000000000000000000, 9.999999999999998224 ) ) ;
#21023=ORIENTED_EDGE ( 'NONE', *, *, #15588, .F. ) ;
#21087=LINE ( 'NONE', #2043, #1360 ) ;
#21163=CARTESIAN_POINT ( 'NONE',  ( 172.7287565553229456, -9.999999999999971578, -36.50000000000000711 ) ) ;
#21199=AXIS2_PLACEMENT_3D ( 'NONE', #29375, #8248, #17848 ) ;
#21227=STYLED_ITEM ( 'NONE', ( #23127 ), #21281 ) ;
#21241=DIRECTION ( 'NONE',  ( -0.000000000000000000, 0.000000000000000000, 1.000000000000000000 ) ) ;
#21261=LINE ( 'NONE', #18822, #8602 ) ;
#21265=ORIENTED_EDGE ( 'NONE', *, *, #17365, .T. ) ;
#21269=EDGE_CURVE ( 'NONE', #19490, #10978, #12461, .T. ) ;
#21281=MANIFOLD_SOLID_BREP ( 'Cut-Extrude1', #22883 ) ;
#21305=ADVANCED_FACE ( 'NONE', ( #13800 ), #2090, .T. ) ;
#21306=EDGE_CURVE ( 'NONE', #16265, #10263, #7700, .T. ) ;
#21315=ORIENTED_EDGE ( 'NONE', *, *, #17481, .T. ) ;
#21322=EDGE_LOOP ( 'NONE', ( #2808, #12916, #3338, #21023 ) ) ;
#21331=EDGE_CURVE ( 'NONE', #25891, #30082, #24165, .T. ) ;
#21348=DIRECTION ( 'NONE',  ( 1.000000000000000000, 0.000000000000000000, 0.000000000000000000 ) ) ;
#21357=DIRECTION ( 'NONE',  ( 0.000000000000000000, 0.000000000000000000, 1.000000000000000000 ) ) ;
#21376=FACE_OUTER_BOUND ( 'NONE', #7453, .T. ) ;
#21384=EDGE_CURVE ( 'NONE', #16793, #30188, #23219, .T. ) ;
#21398=ORIENTED_EDGE ( 'NONE', *, *, #6022, .T. ) ;
#21406=DIRECTION ( 'NONE',  ( 1.000000000000000000, 0.000000000000000000, 0.000000000000000000 ) ) ;
#21440=DIRECTION ( 'NONE',  ( -1.000000000000000000, -2.698458740408365879E-16, -0.000000000000000000 ) ) ;
#21466=DIRECTION ( 'NONE',  ( 1.000000000000000000, 0.000000000000000000, 0.000000000000000000 ) ) ;
#21486=LINE ( 'NONE', #27118, #6711 ) ;
#21516=EDGE_CURVE ( 'NONE', #21824, #4884, #27155, .T. ) ;
#21548=FACE_OUTER_BOUND ( 'NONE', #19111, .T. ) ;
#21576=ORIENTED_EDGE ( 'NONE', *, *, #10309, .T. ) ;
#21614=CARTESIAN_POINT ( 'NONE',  ( 0.000000000000000000, 0.000000000000000000, -15.00000000000000000 ) ) ;
#21627=LINE ( 'NONE', #24234, #26125 ) ;
#21650=LINE ( 'NONE', #28422, #9012 ) ;
#21687=LINE ( 'NONE', #24005, #29775 ) ;
#21741=DIRECTION ( 'NONE',  ( 1.000000000000000000, 2.891205793294675861E-16, 0.000000000000000000 ) ) ;
#21744=ORIENTED_EDGE ( 'NONE', *, *, #28241, .F. ) ;
#21763=EDGE_CURVE ( 'NONE', #1338, #20421, #24183, .T. ) ;
#21772=CARTESIAN_POINT ( 'NONE',  ( 120.0000000000000000, -19.99999999999999645, -186.4312945166758482 ) ) ;
#21790=EDGE_CURVE ( 'NONE', #19672, #14318, #5666, .T. ) ;
#21815=AXIS2_PLACEMENT_3D ( 'NONE', #23676, #4900, #14197 ) ;
#21824=VERTEX_POINT ( 'NONE', #29832 ) ;
#21830=ORIENTED_EDGE ( 'NONE', *, *, #12892, .F. ) ;
#21838=VECTOR ( 'NONE', #3973, 1000.000000000000000 ) ;
#21845=EDGE_LOOP ( 'NONE', ( #8019, #4974 ) ) ;
#21889=DIRECTION ( 'NONE',  ( 1.000000000000000000, 0.000000000000000000, 0.000000000000000000 ) ) ;
#21890=LINE ( 'NONE', #26643, #8291 ) ;
#21955=DIRECTION ( 'NONE',  ( 0.5840962589317576503, -0.8116843969807016057, 0.000000000000000000 ) ) ;
#21969=DIRECTION ( 'NONE',  ( 0.000000000000000000, 0.000000000000000000, -1.000000000000000000 ) ) ;
#22002=AXIS2_PLACEMENT_3D ( 'NONE', #24339, #9981, #21741 ) ;
#22011=CARTESIAN_POINT ( 'NONE',  ( -6.499999999999928946, -11.25833024919774417, -18.00000000000000000 ) ) ;
#22029=CYLINDRICAL_SURFACE ( 'NONE', #24974, 9.000000000000007105 ) ;
#22047=AXIS2_PLACEMENT_3D ( 'NONE', #11012, #20470, #25364 ) ;
#22072=DIRECTION ( 'NONE',  ( 1.000000000000000000, -1.840388255087189623E-16, 0.000000000000000000 ) ) ;
#22088=DIRECTION ( 'NONE',  ( 1.000000000000000000, 0.000000000000000000, 0.000000000000000000 ) ) ;
#22089=CIRCLE ( 'NONE', #8911, 1.500000000000001332 ) ;
#22108=ADVANCED_FACE ( 'NONE', ( #20635, #4320 ), #29726, .T. ) ;
#22165=DIRECTION ( 'NONE',  ( -0.000000000000000000, -0.000000000000000000, 1.000000000000000000 ) ) ;
#22185=CARTESIAN_POINT ( 'NONE',  ( 36.04859390953723874, -22.18451583373416014, -36.50100000000000477 ) ) ;
#22255=DIRECTION ( 'NONE',  ( 0.000000000000000000, 0.000000000000000000, 1.000000000000000000 ) ) ;
#22308=ORIENTED_EDGE ( 'NONE', *, *, #11534, .F. ) ;
#22319=CYLINDRICAL_SURFACE ( 'NONE', #9632, 13.00000000000000178 ) ;
#22329=CARTESIAN_POINT ( 'NONE',  ( 119.9999999999999858, -30.00000000000000000, -15.00000000000000000 ) ) ;
#22334=CARTESIAN_POINT ( 'NONE',  ( 37.54859390953724585, -22.18451583373416014, -15.00000000000000000 ) ) ;
#22362=EDGE_CURVE ( 'NONE', #26545, #3816, #15426, .T. ) ;
#22370=VECTOR ( 'NONE', #5255, 1000.000000000000000 ) ;
#22390=DIRECTION ( 'NONE',  ( -0.000000000000000000, -0.000000000000000000, -1.000000000000000000 ) ) ;
#22424=ADVANCED_FACE ( 'NONE', ( #9179 ), #9333, .F. ) ;
#22499=CARTESIAN_POINT ( 'NONE',  ( 0.000000000000000000, 0.000000000000000000, -15.00000000000000000 ) ) ;
#22520=ORIENTED_EDGE ( 'NONE', *, *, #27131, .T. ) ;
#22592=ADVANCED_FACE ( 'NONE', ( #21548 ), #8251, .T. ) ;
#22637=CARTESIAN_POINT ( 'NONE',  ( 13.00000000000000178, 0.000000000000000000, 18.00000000000000000 ) ) ;
#22639=DIRECTION ( 'NONE',  ( 0.000000000000000000, 0.000000000000000000, 1.000000000000000000 ) ) ;
#22640=UNCERTAINTY_MEASURE_WITH_UNIT (LENGTH_MEASURE( 1.000000000000000082E-05 ), #18116, 'distance_accuracy_value', 'NONE');
#22654=ORIENTED_EDGE ( 'NONE', *, *, #28493, .F. ) ;
#22658=DIRECTION ( 'NONE',  ( -0.000000000000000000, 0.000000000000000000, 1.000000000000000000 ) ) ;
#22724=ORIENTED_EDGE ( 'NONE', *, *, #18758, .F. ) ;
#22734=ORIENTED_EDGE ( 'NONE', *, *, #14057, .T. ) ;
#22763=CIRCLE ( 'NONE', #26679, 129.8897274573438381 ) ;
#22793=EDGE_LOOP ( 'NONE', ( #2740, #14339 ) ) ;
#22803=EDGE_CURVE ( 'NONE', #29492, #3119, #2724, .T. ) ;
#22810=CIRCLE ( 'NONE', #26234, 3.000000000000002665 ) ;
#22823=VERTEX_POINT ( 'NONE', #13134 ) ;
#22829=AXIS2_PLACEMENT_3D ( 'NONE', #29826, #27207, #24890 ) ;
#22883=CLOSED_SHELL ( 'NONE', ( #22424, #1410, #29085, #25934, #13478, #4199, #8620, #1477, #21305, #8322, #13224, #30024, #1038, #4099, #20000, #10975, #22592, #22946, #7368, #17372, #18653, #2716, #28800, #8068, #5466, #29923, #5931, #26432, #5716, #6019, #1687, #14235, #16660, #20545, #17994, #15555, #22108, #18797, #5473, #20204, #16136, #683 ) ) ;
#22893=ORIENTED_EDGE ( 'NONE', *, *, #3678, .T. ) ;
#22902=VECTOR ( 'NONE', #10490, 1000.000000000000000 ) ;
#22905=ORIENTED_EDGE ( 'NONE', *, *, #1454, .T. ) ;
#22942=CARTESIAN_POINT ( 'NONE',  ( -16.00000000000017053, 34.64101615137744972, 4.999999999999998224 ) ) ;
#22946=ADVANCED_FACE ( 'NONE', ( #28688, #16440, #4999 ), #28539, .F. ) ;
#22979=CARTESIAN_POINT ( 'NONE',  ( 175.7287565553229456, -4.999999999999970690, 0.5000000000000029976 ) ) ;
#22987=( NAMED_UNIT ( * ) SI_UNIT ( $, .STERADIAN. ) SOLID_ANGLE_UNIT ( ) );
#22990=DIRECTION ( 'NONE',  ( 1.000000000000000000, 0.000000000000000000, 0.000000000000000000 ) ) ;
#23053=CARTESIAN_POINT ( 'NONE',  ( 0.000000000000000000, 0.000000000000000000, 18.00000000000000000 ) ) ;
#23127=PRESENTATION_STYLE_ASSIGNMENT (( #27746 ) ) ;
#23150=VERTEX_POINT ( 'NONE', #15346 ) ;
#23166=EDGE_CURVE ( 'NONE', #29853, #6425, #3234, .T. ) ;
#23219=CIRCLE ( 'NONE', #4203, 5.000000000000000000 ) ;
#23229=CYLINDRICAL_SURFACE ( 'NONE', #28213, 13.00000000000000178 ) ;
#23254=EDGE_CURVE ( 'NONE', #314, #11816, #16875, .T. ) ;
#23260=ORIENTED_EDGE ( 'NONE', *, *, #1207, .T. ) ;
#23311=AXIS2_PLACEMENT_3D ( 'NONE', #14327, #21969, #28731 ) ;
#23318=VECTOR ( 'NONE', #1093, 1000.000000000000000 ) ;
#23334=EDGE_CURVE ( 'NONE', #14318, #19672, #6638, .T. ) ;
#23349=ORIENTED_EDGE ( 'NONE', *, *, #18823, .F. ) ;
#23357=CARTESIAN_POINT ( 'NONE',  ( -12.69484042717385464, 39.89788248176327556, 9.999999999999998224 ) ) ;
#23388=VECTOR ( 'NONE', #28987, 1000.000000000000000 ) ;
#23395=ORIENTED_EDGE ( 'NONE', *, *, #16304, .F. ) ;
#23421=ORIENTED_EDGE ( 'NONE', *, *, #1318, .T. ) ;
#23434=DIRECTION ( 'NONE',  ( 0.000000000000000000, 0.000000000000000000, 1.000000000000000000 ) ) ;
#23442=ORIENTED_EDGE ( 'NONE', *, *, #21790, .F. ) ;
#23446=ORIENTED_EDGE ( 'NONE', *, *, #5192, .T. ) ;
#23465=AXIS2_PLACEMENT_3D ( 'NONE', #26969, #22658, #18066 ) ;
#23491=VECTOR ( 'NONE', #2985, 1000.000000000000000 ) ;
#23505=ORIENTED_EDGE ( 'NONE', *, *, #15257, .T. ) ;
#23521=ORIENTED_EDGE ( 'NONE', *, *, #20924, .T. ) ;
#23564=ORIENTED_EDGE ( 'NONE', *, *, #17707, .T. ) ;
#23568=ORIENTED_EDGE ( 'NONE', *, *, #1581, .F. ) ;
#23570=DIRECTION ( 'NONE',  ( 1.000000000000000000, 0.000000000000000000, 0.000000000000000000 ) ) ;
#23597=EDGE_CURVE ( 'NONE', #19084, #9938, #2745, .T. ) ;
#23676=CARTESIAN_POINT ( 'NONE',  ( 0.000000000000000000, 0.000000000000000000, 9.999999999999998224 ) ) ;
#23698=ORIENTED_EDGE ( 'NONE', *, *, #28910, .F. ) ;
#23732=LINE ( 'NONE', #28350, #22370 ) ;
#23745=FACE_OUTER_BOUND ( 'NONE', #24379, .T. ) ;
#23765=EDGE_CURVE ( 'NONE', #6425, #29853, #2256, .T. ) ;
#23766=CARTESIAN_POINT ( 'NONE',  ( 0.000000000000000000, 0.000000000000000000, -18.00000000000000000 ) ) ;
#23767=ORIENTED_EDGE ( 'NONE', *, *, #21331, .T. ) ;
#23775=VECTOR ( 'NONE', #14051, 1000.000000000000000 ) ;
#23824=ORIENTED_EDGE ( 'NONE', *, *, #6022, .F. ) ;
#23839=AXIS2_PLACEMENT_3D ( 'NONE', #11807, #17002, #383 ) ;
#23862=CYLINDRICAL_SURFACE ( 'NONE', #18537, 129.8897274573438381 ) ;
#23886=LINE ( 'NONE', #11803, #23491 ) ;
#23888=ORIENTED_EDGE ( 'NONE', *, *, #20615, .F. ) ;
#23948=ORIENTED_EDGE ( 'NONE', *, *, #17818, .T. ) ;
#23970=ORIENTED_EDGE ( 'NONE', *, *, #9718, .T. ) ;
#23979=FACE_OUTER_BOUND ( 'NONE', #15674, .T. ) ;
#24005=CARTESIAN_POINT ( 'NONE',  ( 8.000000000000000000, 9.797174393178825657E-16, 18.00000000000000000 ) ) ;
#24061=EDGE_CURVE ( 'NONE', #14415, #25233, #18814, .T. ) ;
#24094=CARTESIAN_POINT ( 'NONE',  ( 63.44486372867152824, -29.99999999999998934, -17.99999999999998934 ) ) ;
#24121=ORIENTED_EDGE ( 'NONE', *, *, #15206, .T. ) ;
#24138=VECTOR ( 'NONE', #18955, 1000.000000000000000 ) ;
#24152=EDGE_LOOP ( 'NONE', ( #6811, #11843 ) ) ;
#24165=CIRCLE ( 'NONE', #11472, 3.000000000000002665 ) ;
#24183=CIRCLE ( 'NONE', #25161, 13.00000000000000178 ) ;
#24195=DIRECTION ( 'NONE',  ( -0.000000000000000000, 0.000000000000000000, 1.000000000000000000 ) ) ;
#24199=DIRECTION ( 'NONE',  ( 1.000000000000000000, 0.000000000000000000, 0.000000000000000000 ) ) ;
#24203=VECTOR ( 'NONE', #28823, 1000.000000000000000 ) ;
#24208=( NAMED_UNIT ( * ) SI_UNIT ( $, .STERADIAN. ) SOLID_ANGLE_UNIT ( ) );
#24217=CARTESIAN_POINT ( 'NONE',  ( 36.04859390953723874, -22.18451583373416014, -15.00000000000000000 ) ) ;
#24234=CARTESIAN_POINT ( 'NONE',  ( -28.20515957282649921, 30.94299554780361206, 4.999999999999998224 ) ) ;
#24244=DIRECTION ( 'NONE',  ( 0.000000000000000000, 0.000000000000000000, -1.000000000000000000 ) ) ;
#24265=AXIS2_PLACEMENT_3D ( 'NONE', #25969, #25660, #4750 ) ;
#24298=AXIS2_PLACEMENT_3D ( 'NONE', #10205, #7626, #14632 ) ;
#24300=CARTESIAN_POINT ( 'NONE',  ( 63.44486372867152824, 109.8897274573438096, -186.4312945166758482 ) ) ;
#24339=CARTESIAN_POINT ( 'NONE',  ( 133.7287565553229172, -4.999999999999982236, -33.50000000000000000 ) ) ;
#24352=SURFACE_SIDE_STYLE ('',( #19914 ) ) ;
#24353=CIRCLE ( 'NONE', #27333, 3.000000000000002665 ) ;
#24379=EDGE_LOOP ( 'NONE', ( #27579, #13553 ) ) ;
#24391=DIRECTION ( 'NONE',  ( -0.000000000000000000, -0.000000000000000000, -1.000000000000000000 ) ) ;
#24415=( GEOMETRIC_REPRESENTATION_CONTEXT ( 3 ) GLOBAL_UNCERTAINTY_ASSIGNED_CONTEXT ( ( #22640 ) ) GLOBAL_UNIT_ASSIGNED_CONTEXT ( ( #18116, #27024, #15531 ) ) REPRESENTATION_CONTEXT ( 'NONE', 'WORKASPACE' ) );
#24417=DIRECTION ( 'NONE',  ( 0.000000000000000000, 0.000000000000000000, -1.000000000000000000 ) ) ;
#24431=PRODUCT_CONTEXT ( 'NONE', #16112, 'mechanical' ) ;
#24455=ORIENTED_EDGE ( 'NONE', *, *, #24663, .T. ) ;
#24472=CARTESIAN_POINT ( 'NONE',  ( -20.00000000000017053, 34.64101615137744972, 4.999999999999998224 ) ) ;
#24477=CYLINDRICAL_SURFACE ( 'NONE', #18750, 13.00000000000000178 ) ;
#24487=CARTESIAN_POINT ( 'NONE',  ( 10.55189716074911921, 7.593251366112849787, 4.999999999999998224 ) ) ;
#24520=LINE ( 'NONE', #21772, #23388 ) ;
#24538=VERTEX_POINT ( 'NONE', #1715 ) ;
#24584=DIRECTION ( 'NONE',  ( 1.000000000000000000, 0.000000000000000000, 0.000000000000000000 ) ) ;
#24595=ORIENTED_EDGE ( 'NONE', *, *, #26560, .F. ) ;
#24614=DIRECTION ( 'NONE',  ( 1.000000000000000000, 0.000000000000000000, 0.000000000000000000 ) ) ;
#24619=VERTEX_POINT ( 'NONE', #20910 ) ;
#24642=CARTESIAN_POINT ( 'NONE',  ( 0.000000000000000000, 0.000000000000000000, 15.00000000000000000 ) ) ;
#24653=FILL_AREA_STYLE ('',( #26817 ) ) ;
#24663=EDGE_CURVE ( 'NONE', #25233, #28576, #26196, .T. ) ;
#24703=AXIS2_PLACEMENT_3D ( 'NONE', #10409, #15135, #24614 ) ;
#24707=LINE ( 'NONE', #12788, #22902 ) ;
#24750=VERTEX_POINT ( 'NONE', #19221 ) ;
#24783=FACE_OUTER_BOUND ( 'NONE', #4924, .T. ) ;
#24792=VERTEX_POINT ( 'NONE', #10510 ) ;
#24853=DIRECTION ( 'NONE',  ( 0.000000000000000000, -0.000000000000000000, 1.000000000000000000 ) ) ;
#24860=CIRCLE ( 'NONE', #28796, 13.00000000000000178 ) ;
#24890=DIRECTION ( 'NONE',  ( 1.000000000000000000, 0.000000000000000000, 0.000000000000000000 ) ) ;
#24931=DIRECTION ( 'NONE',  ( -1.000000000000000000, 0.000000000000000000, 0.000000000000000000 ) ) ;
#24932=LINE ( 'NONE', #5325, #25789 ) ;
#24974=AXIS2_PLACEMENT_3D ( 'NONE', #24472, #984, #20032 ) ;
#24991=CARTESIAN_POINT ( 'NONE',  ( 0.000000000000000000, 0.000000000000000000, 4.999999999999997335 ) ) ;
#25069=EDGE_CURVE ( 'NONE', #17347, #14415, #11537, .T. ) ;
#25148=EDGE_CURVE ( 'NONE', #2706, #10096, #22763, .T. ) ;
#25153=CARTESIAN_POINT ( 'NONE',  ( 172.7287565553229456, -4.999999999999970690, -33.50000000000000000 ) ) ;
#25161=AXIS2_PLACEMENT_3D ( 'NONE', #7651, #16955, #8840 ) ;
#25207=ORIENTED_EDGE ( 'NONE', *, *, #7407, .F. ) ;
#25220=CARTESIAN_POINT ( 'NONE',  ( 1.244173783436457737E-15, -5.000000000000017764, 0.000000000000000000 ) ) ;
#25233=VERTEX_POINT ( 'NONE', #19045 ) ;
#25247=CIRCLE ( 'NONE', #14015, 13.00000000000000178 ) ;
#25301=DIRECTION ( 'NONE',  ( 1.000000000000000000, 0.000000000000000000, 0.000000000000000000 ) ) ;
#25316=VECTOR ( 'NONE', #26801, 1000.000000000000000 ) ;
#25326=EDGE_LOOP ( 'NONE', ( #27906, #13076, #28136, #23446 ) ) ;
#25364=DIRECTION ( 'NONE',  ( 1.000000000000000000, 0.000000000000000000, 0.000000000000000000 ) ) ;
#25376=EDGE_CURVE ( 'NONE', #4884, #10508, #21486, .T. ) ;
#25430=EDGE_LOOP ( 'NONE', ( #7875, #28870, #26446, #23824 ) ) ;
#25500=EDGE_LOOP ( 'NONE', ( #762, #18682, #10087, #20858 ) ) ;
#25501=ORIENTED_EDGE ( 'NONE', *, *, #1454, .F. ) ;
#25507=CARTESIAN_POINT ( 'NONE',  ( 133.7287565553229172, -9.999999999999980460, -33.50000000000000000 ) ) ;
#25513=CARTESIAN_POINT ( 'NONE',  ( 0.000000000000000000, 0.000000000000000000, 18.00000000000000000 ) ) ;
#25524=CARTESIAN_POINT ( 'NONE',  ( 133.7287565553229456, -4.999999999999982236, 0.5000000000000029976 ) ) ;
#25541=LINE ( 'NONE', #6933, #1066 ) ;
#25596=FACE_OUTER_BOUND ( 'NONE', #19337, .T. ) ;
#25619=VECTOR ( 'NONE', #1037, 1000.000000000000000 ) ;
#25660=DIRECTION ( 'NONE',  ( -1.226925503391459091E-16, 1.000000000000000000, 0.000000000000000000 ) ) ;
#25670=VECTOR ( 'NONE', #22165, 1000.000000000000000 ) ;
#25746=CIRCLE ( 'NONE', #29707, 49.99999999999998579 ) ;
#25748=LINE ( 'NONE', #11690, #10856 ) ;
#25768=FACE_OUTER_BOUND ( 'NONE', #26559, .T. ) ;
#25789=VECTOR ( 'NONE', #2455, 1000.000000000000000 ) ;
#25802=VERTEX_POINT ( 'NONE', #5394 ) ;
#25842=CARTESIAN_POINT ( 'NONE',  ( 0.000000000000000000, 0.000000000000000000, 4.999999999999998224 ) ) ;
#25854=ORIENTED_EDGE ( 'NONE', *, *, #24663, .F. ) ;
#25882=( GEOMETRIC_REPRESENTATION_CONTEXT ( 3 ) GLOBAL_UNCERTAINTY_ASSIGNED_CONTEXT ( ( #11026 ) ) GLOBAL_UNIT_ASSIGNED_CONTEXT ( ( #26354, #28977, #24208 ) ) REPRESENTATION_CONTEXT ( 'NONE', 'WORKASPACE' ) );
#25891=VERTEX_POINT ( 'NONE', #13002 ) ;
#25895=ORIENTED_EDGE ( 'NONE', *, *, #4949, .F. ) ;
#25920=DIRECTION ( 'NONE',  ( 0.000000000000000000, 0.000000000000000000, 1.000000000000000000 ) ) ;
#25922=ORIENTED_EDGE ( 'NONE', *, *, #4980, .T. ) ;
#25934=ADVANCED_FACE ( 'NONE', ( #5844 ), #22319, .T. ) ;
#25963=ORIENTED_EDGE ( 'NONE', *, *, #1552, .F. ) ;
#25969=CARTESIAN_POINT ( 'NONE',  ( 63.44486372867149981, -20.00000000000000355, -186.4312945166758482 ) ) ;
#25987=UNCERTAINTY_MEASURE_WITH_UNIT (LENGTH_MEASURE( 1.000000000000000082E-05 ), #18544, 'distance_accuracy_value', 'NONE');
#25998=DIRECTION ( 'NONE',  ( 1.000000000000000000, 0.000000000000000000, 0.000000000000000000 ) ) ;
#26023=DIRECTION ( 'NONE',  ( -0.000000000000000000, -0.000000000000000000, -1.000000000000000000 ) ) ;
#26045=CIRCLE ( 'NONE', #1182, 5.000000000000000000 ) ;
#26125=VECTOR ( 'NONE', #19487, 1000.000000000000000 ) ;
#26133=AXIS2_PLACEMENT_3D ( 'NONE', #6653, #23434, #13663 ) ;
#26144=EDGE_LOOP ( 'NONE', ( #20381, #8411 ) ) ;
#26170=CARTESIAN_POINT ( 'NONE',  ( 133.7287565553229172, -4.999999999999982236, -36.50000000000000711 ) ) ;
#26182=EDGE_CURVE ( 'NONE', #24619, #2471, #25247, .T. ) ;
#26190=DIRECTION ( 'NONE',  ( 0.000000000000000000, 0.000000000000000000, 1.000000000000000000 ) ) ;
#26196=CIRCLE ( 'NONE', #10572, 3.000000000000002665 ) ;
#26213=LINE ( 'NONE', #7132, #7312 ) ;
#26219=LINE ( 'NONE', #5301, #16130 ) ;
#26222=EDGE_CURVE ( 'NONE', #15024, #29186, #20168, .T. ) ;
#26230=CYLINDRICAL_SURFACE ( 'NONE', #10249, 13.00000000000000178 ) ;
#26234=AXIS2_PLACEMENT_3D ( 'NONE', #7791, #15249, #3668 ) ;
#26237=CARTESIAN_POINT ( 'NONE',  ( 120.0000000000000000, 20.00000000000000355, -17.99999999999998934 ) ) ;
#26246=FACE_OUTER_BOUND ( 'NONE', #18504, .T. ) ;
#26250=VECTOR ( 'NONE', #18900, 1000.000000000000000 ) ;
#26284=EDGE_CURVE ( 'NONE', #16077, #11753, #16452, .T. ) ;
#26302=CIRCLE ( 'NONE', #6796, 13.00000000000000178 ) ;
#26325=PLANE ( 'NONE',  #20632 ) ;
#26335=CARTESIAN_POINT ( 'NONE',  ( 172.7287565553229456, -9.999999999999971578, 0.5000000000000029976 ) ) ;
#26347=LINE ( 'NONE', #14562, #24203 ) ;
#26354=( LENGTH_UNIT ( ) NAMED_UNIT ( * ) SI_UNIT ( .MILLI., .METRE. ) );
#26432=ADVANCED_FACE ( 'NONE', ( #21376 ), #18643, .T. ) ;
#26446=ORIENTED_EDGE ( 'NONE', *, *, #27767, .F. ) ;
#26492=CARTESIAN_POINT ( 'NONE',  ( -20.00000000000017053, 34.64101615137744972, 4.999999999999998224 ) ) ;
#26515=DIRECTION ( 'NONE',  ( 0.000000000000000000, 0.000000000000000000, 1.000000000000000000 ) ) ;
#26545=VERTEX_POINT ( 'NONE', #12815 ) ;
#26559=EDGE_LOOP ( 'NONE', ( #11606, #23260, #27304, #22724 ) ) ;
#26560=EDGE_CURVE ( 'NONE', #15160, #25802, #22810, .T. ) ;
#26593=CARTESIAN_POINT ( 'NONE',  ( 0.000000000000000000, 0.000000000000000000, -15.00000000000000000 ) ) ;
#26597=EDGE_CURVE ( 'NONE', #10096, #27716, #17099, .T. ) ;
#26626=EDGE_LOOP ( 'NONE', ( #16790, #18282 ) ) ;
#26643=CARTESIAN_POINT ( 'NONE',  ( 160.0000000000000000, -10.00000000000000000, -186.4312945166758482 ) ) ;
#26648=ORIENTED_EDGE ( 'NONE', *, *, #1762, .T. ) ;
#26679=AXIS2_PLACEMENT_3D ( 'NONE', #4417, #16449, #18444 ) ;
#26699=AXIS2_PLACEMENT_3D ( 'NONE', #2360, #4928, #21406 ) ;
#26752=ORIENTED_EDGE ( 'NONE', *, *, #9628, .F. ) ;
#26801=DIRECTION ( 'NONE',  ( 0.000000000000000000, 0.000000000000000000, 1.000000000000000000 ) ) ;
#26813=DIRECTION ( 'NONE',  ( 2.908569913943825554E-16, -1.000000000000000000, -0.000000000000000000 ) ) ;
#26817=FILL_AREA_STYLE_COLOUR ( '', #6385 ) ;
#26821=AXIS2_PLACEMENT_3D ( 'NONE', #28874, #1064, #17514 ) ;
#26828=EDGE_CURVE ( 'NONE', #13148, #15024, #3831, .T. ) ;
#26830=DIRECTION ( 'NONE',  ( -1.840388255087189623E-16, -1.000000000000000000, 0.000000000000000000 ) ) ;
#26856=EDGE_CURVE ( 'NONE', #379, #29186, #6417, .T. ) ;
#26917=ORIENTED_EDGE ( 'NONE', *, *, #27131, .F. ) ;
#26926=EDGE_CURVE ( 'NONE', #8342, #20109, #5165, .T. ) ;
#26969=CARTESIAN_POINT ( 'NONE',  ( 0.000000000000000000, 0.000000000000000000, 4.999999999999998224 ) ) ;
#27024=( NAMED_UNIT ( * ) PLANE_ANGLE_UNIT ( ) SI_UNIT ( $, .RADIAN. ) );
#27042=EDGE_CURVE ( 'NONE', #4884, #17347, #9576, .T. ) ;
#27062=ORIENTED_EDGE ( 'NONE', *, *, #26856, .F. ) ;
#27092=CARTESIAN_POINT ( 'NONE',  ( -6.499999999999960032, -11.25833024919772463, -14.99999999999999822 ) ) ;
#27118=CARTESIAN_POINT ( 'NONE',  ( 172.7287565553229456, -4.999999999999970690, -36.50000000000000711 ) ) ;
#27131=EDGE_CURVE ( 'NONE', #12245, #9455, #25746, .T. ) ;
#27155=CIRCLE ( 'NONE', #2276, 3.000000000000002665 ) ;
#27169=VECTOR ( 'NONE', #28788, 1000.000000000000000 ) ;
#27178=CARTESIAN_POINT ( 'NONE',  ( 5.000000000000000000, 6.123233995736766282E-16, 18.00000000000000000 ) ) ;
#27204=AXIS2_PLACEMENT_3D ( 'NONE', #20274, #20576, #8676 ) ;
#27207=DIRECTION ( 'NONE',  ( -0.000000000000000000, 0.000000000000000000, 1.000000000000000000 ) ) ;
#27214=FACE_OUTER_BOUND ( 'NONE', #12014, .T. ) ;
#27294=AXIS2_PLACEMENT_3D ( 'NONE', #20084, #19621, #10619 ) ;
#27304=ORIENTED_EDGE ( 'NONE', *, *, #20371, .T. ) ;
#27314=VECTOR ( 'NONE', #29716, 1000.000000000000114 ) ;
#27333=AXIS2_PLACEMENT_3D ( 'NONE', #11705, #7588, #7140 ) ;
#27335=VECTOR ( 'NONE', #14212, 1000.000000000000000 ) ;
#27350=AXIS2_PLACEMENT_3D ( 'NONE', #10134, #9836, #3000 ) ;
#27404=CYLINDRICAL_SURFACE ( 'NONE', #14721, 8.000000000000000000 ) ;
#27480=CARTESIAN_POINT ( 'NONE',  ( 0.000000000000000000, 0.000000000000000000, -18.00000000000000000 ) ) ;
#27535=ORIENTED_EDGE ( 'NONE', *, *, #21763, .T. ) ;
#27540=DIRECTION ( 'NONE',  ( 1.000000000000000000, 0.000000000000000000, 0.000000000000000000 ) ) ;
#27579=ORIENTED_EDGE ( 'NONE', *, *, #21269, .F. ) ;
#27584=DIRECTION ( 'NONE',  ( 0.000000000000000000, 0.000000000000000000, -1.000000000000000000 ) ) ;
#27604=ORIENTED_EDGE ( 'NONE', *, *, #27042, .T. ) ;
#27618=EDGE_CURVE ( 'NONE', #19921, #29111, #11138, .T. ) ;
#27695=CIRCLE ( 'NONE', #16426, 40.00000000000000711 ) ;
#27716=VERTEX_POINT ( 'NONE', #16551 ) ;
#27746=SURFACE_STYLE_USAGE ( .BOTH. , #9216 ) ;
#27748=CARTESIAN_POINT ( 'NONE',  ( 36.04859390953723874, -22.18451583373416014, -15.00000000000000000 ) ) ;
#27767=EDGE_CURVE ( 'NONE', #4943, #8020, #23732, .T. ) ;
#27823=PRODUCT_DEFINITION_FORMATION_WITH_SPECIFIED_SOURCE ( 'ANY', '', #1575, .NOT_KNOWN. ) ;
#27834=ORIENTED_EDGE ( 'NONE', *, *, #25148, .T. ) ;
#27841=VERTEX_POINT ( 'NONE', #22334 ) ;
#27883=ORIENTED_EDGE ( 'NONE', *, *, #27618, .F. ) ;
#27900=EDGE_CURVE ( 'NONE', #9938, #19629, #10871, .T. ) ;
#27906=ORIENTED_EDGE ( 'NONE', *, *, #15331, .F. ) ;
#27921=FACE_OUTER_BOUND ( 'NONE', #1968, .T. ) ;
#27938=EDGE_CURVE ( 'NONE', #29492, #3816, #1139, .T. ) ;
#27954=CARTESIAN_POINT ( 'NONE',  ( 120.0000000000000000, -19.99999999999999645, -15.00000000000000000 ) ) ;
#27961=AXIS2_PLACEMENT_3D ( 'NONE', #21008, #11533, #25301 ) ;
#27975=ORIENTED_EDGE ( 'NONE', *, *, #489, .F. ) ;
#27999=DIRECTION ( 'NONE',  ( 1.000000000000000000, 0.000000000000000000, 0.000000000000000000 ) ) ;
#28000=CARTESIAN_POINT ( 'NONE',  ( 175.7287565553229456, -4.999999999999970690, -33.50000000000000000 ) ) ;
#28016=DIRECTION ( 'NONE',  ( 2.908569913943825554E-16, -1.000000000000000000, 0.000000000000000000 ) ) ;
#28045=FILL_AREA_STYLE_COLOUR ( '', #28595 ) ;
#28079=EDGE_LOOP ( 'NONE', ( #14333, #22308 ) ) ;
#28087=CARTESIAN_POINT ( 'NONE',  ( 0.000000000000000000, 0.000000000000000000, 15.00000000000000000 ) ) ;
#28100=EDGE_CURVE ( 'NONE', #17512, #21824, #18655, .T. ) ;
#28104=ADVANCED_BREP_SHAPE_REPRESENTATION ( '', ( #21281, #13190 ), #24415 ) ;
#28110=DIRECTION ( 'NONE',  ( 0.000000000000000000, 0.000000000000000000, 1.000000000000000000 ) ) ;
#28136=ORIENTED_EDGE ( 'NONE', *, *, #4949, .T. ) ;
#28213=AXIS2_PLACEMENT_3D ( 'NONE', #7212, #16206, #27999 ) ;
#28230=DIRECTION ( 'NONE',  ( 1.000000000000000000, 0.000000000000000000, 0.000000000000000000 ) ) ;
#28241=EDGE_CURVE ( 'NONE', #19084, #23150, #21687, .T. ) ;
#28255=CARTESIAN_POINT ( 'NONE',  ( 130.7287565553229172, -4.999999999999983125, -36.50000000000000711 ) ) ;
#28262=VECTOR ( 'NONE', #15604, 1000.000000000000000 ) ;
#28271=ORIENTED_EDGE ( 'NONE', *, *, #7811, .T. ) ;
#28281=DIRECTION ( 'NONE',  ( -0.000000000000000000, -0.000000000000000000, -1.000000000000000000 ) ) ;
#28296=CIRCLE ( 'NONE', #10195, 40.00000000000000711 ) ;
#28339=DIRECTION ( 'NONE',  ( 0.000000000000000000, 0.000000000000000000, 1.000000000000000000 ) ) ;
#28350=CARTESIAN_POINT ( 'NONE',  ( 63.44486372867152824, -29.99999999999998934, -15.00000000000000000 ) ) ;
#28376=EDGE_LOOP ( 'NONE', ( #3251, #4285, #22905, #27975 ) ) ;
#28398=FACE_OUTER_BOUND ( 'NONE', #8852, .T. ) ;
#28414=FACE_OUTER_BOUND ( 'NONE', #11936, .T. ) ;
#28422=CARTESIAN_POINT ( 'NONE',  ( 63.44486372867149981, -20.00000000000003197, -186.4312945166758482 ) ) ;
#28423=AXIS2_PLACEMENT_3D ( 'NONE', #25220, #2035, #4153 ) ;
#28458=LINE ( 'NONE', #28765, #24138 ) ;
#28493=EDGE_CURVE ( 'NONE', #3119, #379, #17401, .T. ) ;
#28504=ORIENTED_EDGE ( 'NONE', *, *, #28493, .T. ) ;
#28525=ORIENTED_EDGE ( 'NONE', *, *, #17481, .F. ) ;
#28532=CARTESIAN_POINT ( 'NONE',  ( 119.9999999999999858, -30.00000000000000000, -17.99999999999998934 ) ) ;
#28538=CARTESIAN_POINT ( 'NONE',  ( -11.85189716074913058, -5.341585316273319783, 9.999999999999998224 ) ) ;
#28539=PLANE ( 'NONE',  #12024 ) ;
#28576=VERTEX_POINT ( 'NONE', #20737 ) ;
#28595=COLOUR_RGB ( '', 0.66274510, 0.83137255, 0.94901961) ;
#28649=DIRECTION ( 'NONE',  ( 2.698458740408365879E-16, -1.000000000000000000, 0.000000000000000000 ) ) ;
#28688=FACE_BOUND ( 'NONE', #17146, .T. ) ;
#28696=CARTESIAN_POINT ( 'NONE',  ( 120.0000000000000000, 20.00000000000000355, -15.00000000000000000 ) ) ;
#28731=DIRECTION ( 'NONE',  ( -1.000000000000000000, 0.000000000000000000, 0.000000000000000000 ) ) ;
#28765=CARTESIAN_POINT ( 'NONE',  ( -5.000000000000000000, 0.000000000000000000, 18.00000000000000000 ) ) ;
#28769=DIRECTION ( 'NONE',  ( 0.000000000000000000, 0.000000000000000000, -1.000000000000000000 ) ) ;
#28788=DIRECTION ( 'NONE',  ( 6.938893903907227392E-16, -0.000000000000000000, 1.000000000000000000 ) ) ;
#28796=AXIS2_PLACEMENT_3D ( 'NONE', #22499, #15609, #11465 ) ;
#28800=ADVANCED_FACE ( 'NONE', ( #2162 ), #9142, .T. ) ;
#28823=DIRECTION ( 'NONE',  ( 0.000000000000000000, 0.000000000000000000, -1.000000000000000000 ) ) ;
#28870=ORIENTED_EDGE ( 'NONE', *, *, #10695, .T. ) ;
#28874=CARTESIAN_POINT ( 'NONE',  ( 0.000000000000000000, 0.000000000000000000, 18.00000000000000000 ) ) ;
#28910=EDGE_CURVE ( 'NONE', #14415, #19921, #14024, .T. ) ;
#28962=DIRECTION ( 'NONE',  ( 1.000000000000000000, 0.000000000000000000, 0.000000000000000000 ) ) ;
#28977=( NAMED_UNIT ( * ) PLANE_ANGLE_UNIT ( ) SI_UNIT ( $, .RADIAN. ) );
#28987=DIRECTION ( 'NONE',  ( 0.000000000000000000, 0.000000000000000000, 1.000000000000000000 ) ) ;
#29009=DIRECTION ( 'NONE',  ( -1.000000000000000000, 0.000000000000000000, 0.000000000000000000 ) ) ;
#29085=ADVANCED_FACE ( 'NONE', ( #25596 ), #127, .T. ) ;
#29108=FACE_OUTER_BOUND ( 'NONE', #1444, .T. ) ;
#29111=VERTEX_POINT ( 'NONE', #19182 ) ;
#29162=CARTESIAN_POINT ( 'NONE',  ( -13.00000000000000178, 0.000000000000000000, -15.00000000000000000 ) ) ;
#29168=EDGE_CURVE ( 'NONE', #22823, #13441, #24353, .T. ) ;
#29181=ORIENTED_EDGE ( 'NONE', *, *, #5500, .T. ) ;
#29186=VERTEX_POINT ( 'NONE', #28538 ) ;
#29231=CIRCLE ( 'NONE', #27294, 13.00000000000000178 ) ;
#29264=FACE_OUTER_BOUND ( 'NONE', #21322, .T. ) ;
#29268=DIRECTION ( 'NONE',  ( 1.000000000000000000, 0.000000000000000000, 0.000000000000000000 ) ) ;
#29281=ORIENTED_EDGE ( 'NONE', *, *, #27767, .T. ) ;
#29332=ORIENTED_EDGE ( 'NONE', *, *, #22362, .F. ) ;
#29352=VERTEX_POINT ( 'NONE', #5455 ) ;
#29369=ORIENTED_EDGE ( 'NONE', *, *, #11245, .F. ) ;
#29375=CARTESIAN_POINT ( 'NONE',  ( 130.7287565553229456, -4.999999999999983125, 3.500000000000003109 ) ) ;
#29492=VERTEX_POINT ( 'NONE', #2095 ) ;
#29494=AXIS2_PLACEMENT_3D ( 'NONE', #17363, #7913, #21955 ) ;
#29522=DIRECTION ( 'NONE',  ( -1.000000000000000000, 0.000000000000000000, 0.000000000000000000 ) ) ;
#29524=CARTESIAN_POINT ( 'NONE',  ( -8.000000000000000000, 0.000000000000000000, -15.00000000000000355 ) ) ;
#29555=VECTOR ( 'NONE', #7808, 1000.000000000000000 ) ;
#29576=CARTESIAN_POINT ( 'NONE',  ( 120.0000000000000000, 20.00000000000000355, -186.4312945166758482 ) ) ;
#29588=ORIENTED_EDGE ( 'NONE', *, *, #21763, .F. ) ;
#29595=VECTOR ( 'NONE', #24417, 1000.000000000000000 ) ;
#29601=MECHANICAL_DESIGN_GEOMETRIC_PRESENTATION_REPRESENTATION('',(#21227),#3209);
#29707=AXIS2_PLACEMENT_3D ( 'NONE', #26237, #24391, #5317 ) ;
#29716=DIRECTION ( 'NONE',  ( 0.5840962589317576503, -0.8116843969807016057, 0.000000000000000000 ) ) ;
#29726=PLANE ( 'NONE',  #11522 ) ;
#29772=CARTESIAN_POINT ( 'NONE',  ( 63.44486372867152824, 109.8897274573438096, -17.99999999999998934 ) ) ;
#29775=VECTOR ( 'NONE', #16506, 1000.000000000000000 ) ;
#29798=LINE ( 'NONE', #27178, #2978 ) ;
#29808=CARTESIAN_POINT ( 'NONE',  ( 0.000000000000000000, 0.000000000000000000, -18.00000000000000000 ) ) ;
#29817=EDGE_LOOP ( 'NONE', ( #837, #23505, #11488, #10907 ) ) ;
#29819=ORIENTED_EDGE ( 'NONE', *, *, #10695, .F. ) ;
#29826=CARTESIAN_POINT ( 'NONE',  ( -20.00000000000017053, 34.64101615137744972, 9.999999999999998224 ) ) ;
#29832=CARTESIAN_POINT ( 'NONE',  ( 175.7287565553229456, -4.999999999999970690, -33.50000000000000000 ) ) ;
#29853=VERTEX_POINT ( 'NONE', #603 ) ;
#29923=ADVANCED_FACE ( 'NONE', ( #28414 ), #4718, .T. ) ;
#29963=EDGE_LOOP ( 'NONE', ( #23888, #20151, #434, #20852 ) ) ;
#30009=FACE_OUTER_BOUND ( 'NONE', #29963, .T. ) ;
#30017=ORIENTED_EDGE ( 'NONE', *, *, #5192, .F. ) ;
#30018=CARTESIAN_POINT ( 'NONE',  ( 10.55189716074911921, 7.593251366112849787, 4.999999999999998224 ) ) ;
#30024=ADVANCED_FACE ( 'NONE', ( #15220, #19352 ), #5329, .T. ) ;
#30031=ORIENTED_EDGE ( 'NONE', *, *, #29168, .T. ) ;
#30062=DIRECTION ( 'NONE',  ( 1.000000000000000000, 0.000000000000000000, 0.000000000000000000 ) ) ;
#30082=VERTEX_POINT ( 'NONE', #1067 ) ;
#30121=CYLINDRICAL_SURFACE ( 'NONE', #3053, 5.000000000000000000 ) ;
#30185=DIRECTION ( 'NONE',  ( 0.5840962589317576503, -0.8116843969807016057, 0.000000000000000000 ) ) ;
#30188=VERTEX_POINT ( 'NONE', #3798 ) ;
#30227=DIRECTION ( 'NONE',  ( -2.908569913943825554E-16, 1.000000000000000000, 0.000000000000000000 ) ) ;
#30235=PLANE ( 'NONE',  #14088 ) ;
#30257=EDGE_CURVE ( 'NONE', #30188, #8805, #29798, .T. ) ;
ENDSEC;
END-ISO-10303-21;
